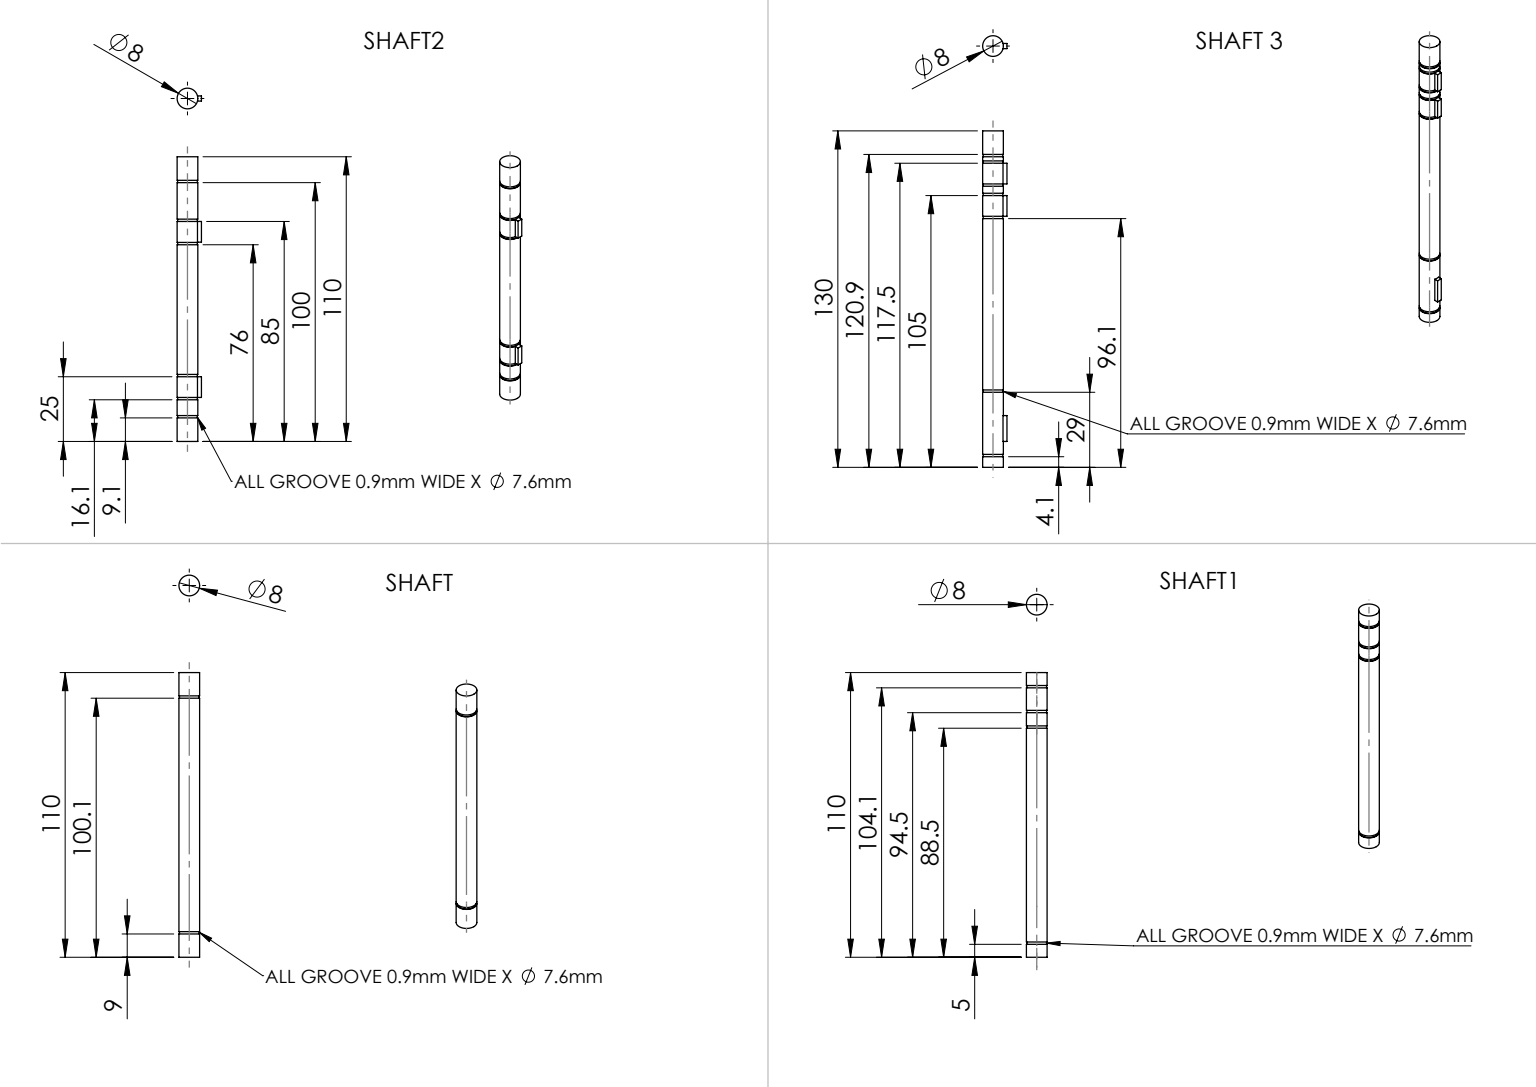
ISO-10303-21;
HEADER;
FILE_DESCRIPTION (('STEP AP214'),
    '1' );
FILE_NAME ('shaft 3.step',
    '2026-09-28T15:49:00',
    ( '' ),
    ( '' ),
    'SwSTEP 2.0',
    'SolidWorks 2026',
    '' );
FILE_SCHEMA (( 'AUTOMOTIVE_DESIGN' ));
ENDSEC;

DATA;
#35=DIRECTION ( 'NONE',  ( 0.000000000000000000, 0.000000000000000000, 1.000000000000000000 ) ) ;
#45=CIRCLE ( 'NONE', #32841, 4.000000000000000000 ) ;
#49=ORIENTED_EDGE ( 'NONE', *, *, #14010, .T. ) ;
#53=ORIENTED_EDGE ( 'NONE', *, *, #22089, .T. ) ;
#63=EDGE_CURVE ( 'NONE', #29341, #31925, #15789, .T. ) ;
#64=FACE_BOUND ( 'NONE', #18708, .T. ) ;
#78=CARTESIAN_POINT ( 'NONE',  ( 0.000000000000000000, 0.000000000000000000, -52.50000000000000000 ) ) ;
#94=EDGE_LOOP ( 'NONE', ( #19216, #26930 ) ) ;
#103=DIRECTION ( 'NONE',  ( 0.000000000000000000, 0.000000000000000000, 1.000000000000000000 ) ) ;
#158=DIRECTION ( 'NONE',  ( 1.000000000000000000, 0.000000000000000000, 0.000000000000000000 ) ) ;
#161=AXIS2_PLACEMENT_3D ( 'NONE', #25822, #31910, #29039 ) ;
#163=AXIS2_PLACEMENT_3D ( 'NONE', #32400, #32750, #18355 ) ;
#170=EDGE_LOOP ( 'NONE', ( #28975, #27946, #5714, #16850, #18978 ) ) ;
#184=ORIENTED_EDGE ( 'NONE', *, *, #5407, .T. ) ;
#201=DIRECTION ( 'NONE',  ( 0.000000000000000000, 0.000000000000000000, -1.000000000000000000 ) ) ;
#243=UNCERTAINTY_MEASURE_WITH_UNIT (LENGTH_MEASURE( 1.000000000000000082E-05 ), #22968, 'distance_accuracy_value', 'NONE');
#244=FACE_BOUND ( 'NONE', #10635, .T. ) ;
#313=EDGE_CURVE ( 'NONE', #20125, #14882, #23736, .T. ) ;
#334=VERTEX_POINT ( 'NONE', #10530 ) ;
#363=VECTOR ( 'NONE', #32529, 1000.000000000000000 ) ;
#379=CIRCLE ( 'NONE', #19345, 3.799999999999999822 ) ;
#397=VECTOR ( 'NONE', #13640, 1000.000000000000000 ) ;
#407=ORIENTED_EDGE ( 'NONE', *, *, #33311, .T. ) ;
#422=AXIS2_PLACEMENT_3D ( 'NONE', #13815, #3025, #22085 ) ;
#445=ORIENTED_EDGE ( 'NONE', *, *, #2012, .T. ) ;
#457=AXIS2_PLACEMENT_3D ( 'NONE', #23375, #28612, #18143 ) ;
#529=VERTEX_POINT ( 'NONE', #3676 ) ;
#548=DIRECTION ( 'NONE',  ( 0.000000000000000000, 0.000000000000000000, -1.000000000000000000 ) ) ;
#559=CARTESIAN_POINT ( 'NONE',  ( 0.000000000000000000, 0.000000000000000000, 36.00000000000000000 ) ) ;
#569=ORIENTED_EDGE ( 'NONE', *, *, #1551, .F. ) ;
#602=AXIS2_PLACEMENT_3D ( 'NONE', #22892, #9216, #15491 ) ;
#667=EDGE_CURVE ( 'NONE', #19003, #35092, #26350, .T. ) ;
#681=ADVANCED_FACE ( 'NONE', ( #6712 ), #12122, .T. ) ;
#708=VERTEX_POINT ( 'NONE', #10129 ) ;
#719=FACE_BOUND ( 'NONE', #18642, .T. ) ;
#759=EDGE_CURVE ( 'NONE', #1825, #2615, #29234, .T. ) ;
#762=EDGE_LOOP ( 'NONE', ( #23017, #33225, #3692, #5978 ) ) ;
#799=AXIS2_PLACEMENT_3D ( 'NONE', #2899, #3428, #30949 ) ;
#875=DIRECTION ( 'NONE',  ( -1.000000000000000000, 0.000000000000000000, 0.000000000000000000 ) ) ;
#891=VERTEX_POINT ( 'NONE', #10669 ) ;
#925=EDGE_CURVE ( 'NONE', #1732, #8675, #21625, .T. ) ;
#926=ADVANCED_FACE ( 'NONE', ( #19110 ), #21813, .F. ) ;
#939=DIRECTION ( 'NONE',  ( 0.000000000000000000, 0.000000000000000000, -1.000000000000000000 ) ) ;
#946=VECTOR ( 'NONE', #32460, 1000.000000000000000 ) ;
#971=CARTESIAN_POINT ( 'NONE',  ( -4.000000000000000000, 0.000000000000000000, 65.00000000000000000 ) ) ;
#1057=AXIS2_PLACEMENT_3D ( 'NONE', #25207, #11856, #34016 ) ;
#1062=CARTESIAN_POINT ( 'NONE',  ( -4.000000000000000000, 0.000000000000000000, -40.00000000000000711 ) ) ;
#1089=EDGE_CURVE ( 'NONE', #18547, #14157, #25484, .T. ) ;
#1104=EDGE_CURVE ( 'NONE', #9474, #16728, #8811, .T. ) ;
#1115=CARTESIAN_POINT ( 'NONE',  ( 4.000000000000000000, 4.898587196589412829E-16, 55.00000000000000711 ) ) ;
#1131=ORIENTED_EDGE ( 'NONE', *, *, #8517, .T. ) ;
#1185=EDGE_LOOP ( 'NONE', ( #21946, #29122, #4099, #24705 ) ) ;
#1199=ORIENTED_EDGE ( 'NONE', *, *, #32627, .T. ) ;
#1200=ORIENTED_EDGE ( 'NONE', *, *, #17363, .T. ) ;
#1212=FACE_BOUND ( 'NONE', #25738, .T. ) ;
#1243=PLANE ( 'NONE',  #13482 ) ;
#1250=DIRECTION ( 'NONE',  ( 1.000000000000000000, 0.000000000000000000, 0.000000000000000000 ) ) ;
#1290=FACE_OUTER_BOUND ( 'NONE', #13785, .T. ) ;
#1308=CARTESIAN_POINT ( 'NONE',  ( 5.400000000000085620, -1.000000000000049516, -44.50000000000000000 ) ) ;
#1386=ADVANCED_FACE ( 'NONE', ( #10817 ), #35486, .F. ) ;
#1408=LINE ( 'NONE', #20464, #3158 ) ;
#1411=DIRECTION ( 'NONE',  ( 1.000000000000000000, 0.000000000000000000, 0.000000000000000000 ) ) ;
#1422=ORIENTED_EDGE ( 'NONE', *, *, #667, .F. ) ;
#1425=CARTESIAN_POINT ( 'NONE',  ( 0.000000000000000000, 0.000000000000000000, -53.39999999999999858 ) ) ;
#1483=AXIS2_PLACEMENT_3D ( 'NONE', #27788, #939, #24901 ) ;
#1511=LINE ( 'NONE', #12493, #7664 ) ;
#1546=VERTEX_POINT ( 'NONE', #35138 ) ;
#1551=EDGE_CURVE ( 'NONE', #20125, #33416, #27029, .T. ) ;
#1555=CARTESIAN_POINT ( 'NONE',  ( 9.714451465470119729E-14, 0.9999999999999870104, -52.50000000000000000 ) ) ;
#1570=CARTESIAN_POINT ( 'NONE',  ( 3.799999999999999822, 0.000000000000000000, -43.60000000000000142 ) ) ;
#1604=DIRECTION ( 'NONE',  ( -1.000000000000000000, 1.110223024625156540E-16, 0.000000000000000000 ) ) ;
#1608=VECTOR ( 'NONE', #26480, 1000.000000000000000 ) ;
#1627=ADVANCED_FACE ( 'NONE', ( #16893 ), #33129, .T. ) ;
#1680=CARTESIAN_POINT ( 'NONE',  ( 0.000000000000000000, 0.000000000000000000, -44.50000000000000000 ) ) ;
#1708=EDGE_CURVE ( 'NONE', #10690, #33549, #14030, .T. ) ;
#1726=PLANE ( 'NONE',  #34542 ) ;
#1732=VERTEX_POINT ( 'NONE', #11857 ) ;
#1792=ADVANCED_FACE ( 'NONE', ( #15077 ), #1243, .F. ) ;
#1804=CARTESIAN_POINT ( 'NONE',  ( 0.000000000000000000, 0.000000000000000000, -65.00000000000000000 ) ) ;
#1825=VERTEX_POINT ( 'NONE', #31305 ) ;
#1844=( NAMED_UNIT ( * ) SI_UNIT ( $, .STERADIAN. ) SOLID_ANGLE_UNIT ( ) );
#1850=VERTEX_POINT ( 'NONE', #26266 ) ;
#1869=CIRCLE ( 'NONE', #16244, 4.000000000000000000 ) ;
#1889=DIRECTION ( 'NONE',  ( 0.000000000000000000, 0.000000000000000000, 1.000000000000000000 ) ) ;
#1939=DIRECTION ( 'NONE',  ( -1.000000000000000000, 0.000000000000000000, 0.000000000000000000 ) ) ;
#1949=DIRECTION ( 'NONE',  ( 0.000000000000000000, 0.000000000000000000, 1.000000000000000000 ) ) ;
#1997=EDGE_CURVE ( 'NONE', #15000, #23250, #32199, .T. ) ;
#2012=EDGE_CURVE ( 'NONE', #5174, #9474, #13646, .T. ) ;
#2210=VERTEX_POINT ( 'NONE', #8932 ) ;
#2215=ORIENTED_EDGE ( 'NONE', *, *, #19628, .T. ) ;
#2274=CARTESIAN_POINT ( 'NONE',  ( -3.799999999999999822, 4.653657836759942730E-16, 36.00000000000000000 ) ) ;
#2286=ADVANCED_FACE ( 'NONE', ( #20615 ), #34149, .T. ) ;
#2290=CYLINDRICAL_SURFACE ( 'NONE', #32641, 4.000000000000000000 ) ;
#2299=FACE_OUTER_BOUND ( 'NONE', #28981, .T. ) ;
#2300=EDGE_CURVE ( 'NONE', #17838, #10539, #13512, .T. ) ;
#2305=EDGE_LOOP ( 'NONE', ( #16724, #26388, #32363, #12762 ) ) ;
#2311=AXIS2_PLACEMENT_3D ( 'NONE', #28801, #12776, #4327 ) ;
#2355=VECTOR ( 'NONE', #11953, 1000.000000000000000 ) ;
#2357=DIRECTION ( 'NONE',  ( -1.000000000000000000, 0.000000000000000000, 0.000000000000000000 ) ) ;
#2394=CIRCLE ( 'NONE', #19595, 4.000000000000000000 ) ;
#2432=CARTESIAN_POINT ( 'NONE',  ( -4.000000000000000000, 0.000000000000000000, -40.89999999999999858 ) ) ;
#2504=VERTEX_POINT ( 'NONE', #21694 ) ;
#2506=EDGE_LOOP ( 'NONE', ( #10673, #1199, #407, #34930 ) ) ;
#2513=ORIENTED_EDGE ( 'NONE', *, *, #34592, .F. ) ;
#2528=CARTESIAN_POINT ( 'NONE',  ( 5.400000000000085620, -1.000000000000049516, -32.00000000000000000 ) ) ;
#2537=ORIENTED_EDGE ( 'NONE', *, *, #1089, .T. ) ;
#2547=AXIS2_PLACEMENT_3D ( 'NONE', #16252, #21483, #32476 ) ;
#2576=AXIS2_PLACEMENT_3D ( 'NONE', #11160, #33643, #875 ) ;
#2603=DIRECTION ( 'NONE',  ( -0.000000000000000000, 0.000000000000000000, -1.000000000000000000 ) ) ;
#2615=VERTEX_POINT ( 'NONE', #16277 ) ;
#2620=DIRECTION ( 'NONE',  ( -1.000000000000000000, 0.000000000000000000, 0.000000000000000000 ) ) ;
#2656=AXIS2_PLACEMENT_3D ( 'NONE', #3682, #14632, #19675 ) ;
#2665=AXIS2_PLACEMENT_3D ( 'NONE', #16709, #18893, #16351 ) ;
#2674=LINE ( 'NONE', #29500, #397 ) ;
#2693=VERTEX_POINT ( 'NONE', #11083 ) ;
#2738=ORIENTED_EDGE ( 'NONE', *, *, #27732, .F. ) ;
#2790=LINE ( 'NONE', #12548, #11992 ) ;
#2792=DIRECTION ( 'NONE',  ( -1.000000000000000000, 0.000000000000000000, 0.000000000000000000 ) ) ;
#2793=AXIS2_PLACEMENT_3D ( 'NONE', #9523, #6992, #31309 ) ;
#2847=DIRECTION ( 'NONE',  ( -1.000000000000000000, 0.000000000000000000, 0.000000000000000000 ) ) ;
#2899=CARTESIAN_POINT ( 'NONE',  ( 0.000000000000000000, 0.000000000000000000, -40.89999999999999858 ) ) ;
#2901=EDGE_CURVE ( 'NONE', #13424, #2693, #1511, .T. ) ;
#2935=DIRECTION ( 'NONE',  ( -1.000000000000000000, 0.000000000000000000, 0.000000000000000000 ) ) ;
#3018=DIRECTION ( 'NONE',  ( 1.000000000000000000, -1.110223024625156540E-16, 0.000000000000000000 ) ) ;
#3025=DIRECTION ( 'NONE',  ( 1.110223024625156540E-16, 1.000000000000000000, 0.000000000000000000 ) ) ;
#3048=AXIS2_PLACEMENT_3D ( 'NONE', #11758, #3330, #33731 ) ;
#3086=AXIS2_PLACEMENT_3D ( 'NONE', #9014, #22341, #11712 ) ;
#3125=ORIENTED_EDGE ( 'NONE', *, *, #31259, .T. ) ;
#3136=DIRECTION ( 'NONE',  ( -1.000000000000000000, 8.604228440844963188E-16, 0.000000000000000000 ) ) ;
#3158=VECTOR ( 'NONE', #26077, 1000.000000000000000 ) ;
#3196=PLANE ( 'NONE',  #422 ) ;
#3243=FACE_OUTER_BOUND ( 'NONE', #27570, .T. ) ;
#3268=DIRECTION ( 'NONE',  ( -0.000000000000000000, 0.000000000000000000, -1.000000000000000000 ) ) ;
#3282=VERTEX_POINT ( 'NONE', #30098 ) ;
#3311=AXIS2_PLACEMENT_3D ( 'NONE', #78, #11065, #22035 ) ;
#3328=ADVANCED_FACE ( 'NONE', ( #24167 ), #16388, .T. ) ;
#3330=DIRECTION ( 'NONE',  ( 0.000000000000000000, 0.000000000000000000, -1.000000000000000000 ) ) ;
#3339=CARTESIAN_POINT ( 'NONE',  ( 0.000000000000000000, 0.000000000000000000, 60.90000000000001279 ) ) ;
#3373=CARTESIAN_POINT ( 'NONE',  ( 1.110223024625156540E-13, -1.000000000000042633, -52.50000000000000000 ) ) ;
#3393=PLANE ( 'NONE',  #18283 ) ;
#3400=CYLINDRICAL_SURFACE ( 'NONE', #16840, 4.000000000000000000 ) ;
#3428=DIRECTION ( 'NONE',  ( 0.000000000000000000, 0.000000000000000000, 1.000000000000000000 ) ) ;
#3431=AXIS2_PLACEMENT_3D ( 'NONE', #3458, #30804, #5797 ) ;
#3458=CARTESIAN_POINT ( 'NONE',  ( 0.000000000000000000, 0.000000000000000000, -31.10000000000000142 ) ) ;
#3492=CARTESIAN_POINT ( 'NONE',  ( 3.872983346207517386, -1.000000000000028644, -40.00000000000000711 ) ) ;
#3507=DIRECTION ( 'NONE',  ( -1.000000000000000000, 0.000000000000000000, 0.000000000000000000 ) ) ;
#3549=CARTESIAN_POINT ( 'NONE',  ( 5.400000000000085620, -1.000000000000049516, -32.00000000000000000 ) ) ;
#3558=CARTESIAN_POINT ( 'NONE',  ( -3.799999999999999822, 4.653657836759942730E-16, -40.89999999999999858 ) ) ;
#3580=DIRECTION ( 'NONE',  ( 0.000000000000000000, 0.000000000000000000, -1.000000000000000000 ) ) ;
#3619=AXIS2_PLACEMENT_3D ( 'NONE', #31515, #15279, #17807 ) ;
#3643=ORIENTED_EDGE ( 'NONE', *, *, #15823, .T. ) ;
#3649=ORIENTED_EDGE ( 'NONE', *, *, #4897, .F. ) ;
#3659=EDGE_CURVE ( 'NONE', #32739, #28967, #8206, .T. ) ;
#3669=CARTESIAN_POINT ( 'NONE',  ( 0.000000000000000000, 0.000000000000000000, -53.39999999999999858 ) ) ;
#3676=CARTESIAN_POINT ( 'NONE',  ( 3.799999999999999822, 0.000000000000000000, -53.39999999999999858 ) ) ;
#3682=CARTESIAN_POINT ( 'NONE',  ( 0.000000000000000000, 0.000000000000000000, 60.00000000000000000 ) ) ;
#3687=DIRECTION ( 'NONE',  ( 0.000000000000000000, 0.000000000000000000, -1.000000000000000000 ) ) ;
#3692=ORIENTED_EDGE ( 'NONE', *, *, #7492, .T. ) ;
#3716=VECTOR ( 'NONE', #9190, 1000.000000000000000 ) ;
#3753=CARTESIAN_POINT ( 'NONE',  ( 0.000000000000000000, 0.000000000000000000, -44.50000000000000000 ) ) ;
#3771=CARTESIAN_POINT ( 'NONE',  ( 3.872983346207517386, -1.000000000000028644, 65.00000000000000000 ) ) ;
#3772=CIRCLE ( 'NONE', #11790, 4.000000000000000000 ) ;
#3777=CIRCLE ( 'NONE', #1483, 3.799999999999999822 ) ;
#3790=CARTESIAN_POINT ( 'NONE',  ( 3.872983346207517386, -1.000000000000028644, 45.00000000000000711 ) ) ;
#3805=FACE_OUTER_BOUND ( 'NONE', #2506, .T. ) ;
#3818=ADVANCED_FACE ( 'NONE', ( #32047 ), #18887, .T. ) ;
#3840=AXIS2_PLACEMENT_3D ( 'NONE', #18949, #10329, #35538 ) ;
#3900=CIRCLE ( 'NONE', #3311, 4.000000000000000000 ) ;
#3912=VECTOR ( 'NONE', #31497, 1000.000000000000000 ) ;
#3917=LINE ( 'NONE', #1555, #26870 ) ;
#3965=AXIS2_PLACEMENT_3D ( 'NONE', #10553, #103, #30006 ) ;
#3992=FACE_OUTER_BOUND ( 'NONE', #30123, .T. ) ;
#3997=VERTEX_POINT ( 'NONE', #30578 ) ;
#4033=DIRECTION ( 'NONE',  ( 0.000000000000000000, 0.000000000000000000, -1.000000000000000000 ) ) ;
#4042=PLANE ( 'NONE',  #23335 ) ;
#4046=AXIS2_PLACEMENT_3D ( 'NONE', #8922, #31077, #28028 ) ;
#4050=FACE_OUTER_BOUND ( 'NONE', #30940, .T. ) ;
#4069=ADVANCED_FACE ( 'NONE', ( #9499 ), #28946, .T. ) ;
#4099=ORIENTED_EDGE ( 'NONE', *, *, #1997, .F. ) ;
#4129=FACE_BOUND ( 'NONE', #21760, .T. ) ;
#4166=DIRECTION ( 'NONE',  ( -0.000000000000000000, 0.000000000000000000, -1.000000000000000000 ) ) ;
#4224=DIRECTION ( 'NONE',  ( 0.000000000000000000, 0.000000000000000000, -1.000000000000000000 ) ) ;
#4255=CARTESIAN_POINT ( 'NONE',  ( 0.000000000000000000, 0.000000000000000000, 60.00000000000000000 ) ) ;
#4281=EDGE_CURVE ( 'NONE', #11309, #17651, #27314, .T. ) ;
#4312=CARTESIAN_POINT ( 'NONE',  ( 1.110223024625156540E-13, -1.000000000000042633, -44.50000000000000000 ) ) ;
#4317=DIRECTION ( 'NONE',  ( -0.000000000000000000, 0.000000000000000000, -1.000000000000000000 ) ) ;
#4327=DIRECTION ( 'NONE',  ( -1.000000000000000000, 0.000000000000000000, 0.000000000000000000 ) ) ;
#4366=ORIENTED_EDGE ( 'NONE', *, *, #16719, .F. ) ;
#4389=CARTESIAN_POINT ( 'NONE',  ( 0.000000000000000000, 0.000000000000000000, -40.89999999999999858 ) ) ;
#4431=CIRCLE ( 'NONE', #11305, 3.799999999999999822 ) ;
#4439=LINE ( 'NONE', #10182, #11323 ) ;
#4440=CARTESIAN_POINT ( 'NONE',  ( 0.000000000000000000, 0.000000000000000000, -40.00000000000000000 ) ) ;
#4465=DIRECTION ( 'NONE',  ( 0.000000000000000000, 0.000000000000000000, -1.000000000000000000 ) ) ;
#4475=DIRECTION ( 'NONE',  ( 0.000000000000000000, 0.000000000000000000, -1.000000000000000000 ) ) ;
#4477=VECTOR ( 'NONE', #3136, 1000.000000000000000 ) ;
#4527=DIRECTION ( 'NONE',  ( 0.000000000000000000, 0.000000000000000000, -1.000000000000000000 ) ) ;
#4531=FACE_OUTER_BOUND ( 'NONE', #15351, .T. ) ;
#4558=PRESENTATION_STYLE_ASSIGNMENT (( #26863 ) ) ;
#4630=( NAMED_UNIT ( * ) PLANE_ANGLE_UNIT ( ) SI_UNIT ( $, .RADIAN. ) );
#4645=ORIENTED_EDGE ( 'NONE', *, *, #28476, .T. ) ;
#4652=ORIENTED_EDGE ( 'NONE', *, *, #24673, .F. ) ;
#4663=FACE_OUTER_BOUND ( 'NONE', #2305, .T. ) ;
#4666=CARTESIAN_POINT ( 'NONE',  ( 0.000000000000000000, 0.000000000000000000, -40.89999999999999858 ) ) ;
#4729=ORIENTED_EDGE ( 'NONE', *, *, #30126, .T. ) ;
#4736=ADVANCED_FACE ( 'NONE', ( #22032, #11708 ), #14405, .F. ) ;
#4777=CARTESIAN_POINT ( 'NONE',  ( -4.000000000000000000, 0.000000000000000000, -55.89999999999999858 ) ) ;
#4845=EDGE_CURVE ( 'NONE', #12683, #2615, #22867, .T. ) ;
#4852=ADVANCED_FACE ( 'NONE', ( #27098, #13408 ), #35376, .T. ) ;
#4853=LINE ( 'NONE', #12947, #8691 ) ;
#4884=ADVANCED_FACE ( 'NONE', ( #3992, #23044 ), #14763, .F. ) ;
#4897=EDGE_CURVE ( 'NONE', #28967, #28820, #17816, .T. ) ;
#4898=SURFACE_SIDE_STYLE ('',( #29384 ) ) ;
#4910=AXIS2_PLACEMENT_3D ( 'NONE', #32006, #7345, #24099 ) ;
#4920=ORIENTED_EDGE ( 'NONE', *, *, #2300, .T. ) ;
#5004=AXIS2_PLACEMENT_3D ( 'NONE', #22998, #3580, #14527 ) ;
#5037=ORIENTED_EDGE ( 'NONE', *, *, #17189, .F. ) ;
#5096=VECTOR ( 'NONE', #8374, 1000.000000000000000 ) ;
#5108=ADVANCED_FACE ( 'NONE', ( #5235 ), #21049, .T. ) ;
#5174=VERTEX_POINT ( 'NONE', #22297 ) ;
#5175=AXIS2_PLACEMENT_3D ( 'NONE', #17449, #14748, #18525 ) ;
#5191=CYLINDRICAL_SURFACE ( 'NONE', #29029, 3.799999999999999822 ) ;
#5205=CARTESIAN_POINT ( 'NONE',  ( -3.799999999999999822, 4.653657836759942730E-16, 35.10000000000000142 ) ) ;
#5235=FACE_OUTER_BOUND ( 'NONE', #33749, .T. ) ;
#5242=ORIENTED_EDGE ( 'NONE', *, *, #16113, .T. ) ;
#5263=DIRECTION ( 'NONE',  ( 1.000000000000000000, 0.000000000000000000, 0.000000000000000000 ) ) ;
#5276=DIRECTION ( 'NONE',  ( 1.000000000000000000, 0.000000000000000000, 0.000000000000000000 ) ) ;
#5277=CIRCLE ( 'NONE', #12147, 4.000000000000000000 ) ;
#5282=VERTEX_POINT ( 'NONE', #19582 ) ;
#5286=DIRECTION ( 'NONE',  ( 0.000000000000000000, 0.000000000000000000, -1.000000000000000000 ) ) ;
#5304=LINE ( 'NONE', #16242, #22925 ) ;
#5329=VERTEX_POINT ( 'NONE', #17237 ) ;
#5361=LINE ( 'NONE', #15961, #21056 ) ;
#5362=DIRECTION ( 'NONE',  ( 0.000000000000000000, 0.000000000000000000, -1.000000000000000000 ) ) ;
#5371=ORIENTED_EDGE ( 'NONE', *, *, #14296, .T. ) ;
#5383=CARTESIAN_POINT ( 'NONE',  ( 9.714451465470119729E-14, 0.9999999999999870104, -32.00000000000000000 ) ) ;
#5407=EDGE_CURVE ( 'NONE', #23250, #34581, #1408, .T. ) ;
#5421=AXIS2_PLACEMENT_3D ( 'NONE', #21421, #16185, #29553 ) ;
#5498=EDGE_CURVE ( 'NONE', #21576, #30905, #34005, .T. ) ;
#5512=CARTESIAN_POINT ( 'NONE',  ( 3.799999999999999822, 0.000000000000000000, 60.90000000000001279 ) ) ;
#5528=CYLINDRICAL_SURFACE ( 'NONE', #18245, 3.799999999999999822 ) ;
#5559=ADVANCED_FACE ( 'NONE', ( #10576 ), #5191, .T. ) ;
#5604=CARTESIAN_POINT ( 'NONE',  ( 0.000000000000000000, 0.000000000000000000, 55.00000000000000711 ) ) ;
#5616=EDGE_CURVE ( 'NONE', #32249, #2504, #3772, .T. ) ;
#5652=EDGE_CURVE ( 'NONE', #28820, #8675, #32488, .T. ) ;
#5653=CIRCLE ( 'NONE', #32659, 3.799999999999999822 ) ;
#5692=DIRECTION ( 'NONE',  ( 1.000000000000000000, 0.000000000000000000, 0.000000000000000000 ) ) ;
#5695=ADVANCED_FACE ( 'NONE', ( #13120 ), #21003, .T. ) ;
#5708=EDGE_LOOP ( 'NONE', ( #10243, #32904 ) ) ;
#5714=ORIENTED_EDGE ( 'NONE', *, *, #22916, .T. ) ;
#5738=EDGE_CURVE ( 'NONE', #19012, #12683, #8390, .T. ) ;
#5744=CARTESIAN_POINT ( 'NONE',  ( 0.000000000000000000, 0.000000000000000000, -40.00000000000000000 ) ) ;
#5797=DIRECTION ( 'NONE',  ( -1.000000000000000000, 0.000000000000000000, 0.000000000000000000 ) ) ;
#5873=CYLINDRICAL_SURFACE ( 'NONE', #18776, 4.000000000000000000 ) ;
#5913=DIRECTION ( 'NONE',  ( -1.000000000000000000, 0.000000000000000000, 0.000000000000000000 ) ) ;
#5944=EDGE_LOOP ( 'NONE', ( #18134, #30778, #21079, #31987 ) ) ;
#5962=EDGE_CURVE ( 'NONE', #21809, #12683, #34496, .T. ) ;
#5978=ORIENTED_EDGE ( 'NONE', *, *, #10678, .T. ) ;
#5985=ORIENTED_EDGE ( 'NONE', *, *, #14960, .F. ) ;
#6061=DIRECTION ( 'NONE',  ( 0.000000000000000000, 0.000000000000000000, 1.000000000000000000 ) ) ;
#6063=AXIS2_PLACEMENT_3D ( 'NONE', #6140, #4166, #11888 ) ;
#6065=UNCERTAINTY_MEASURE_WITH_UNIT (LENGTH_MEASURE( 1.000000000000000082E-05 ), #29911, 'distance_accuracy_value', 'NONE');
#6072=SHAPE_DEFINITION_REPRESENTATION ( #23625, #18063 ) ;
#6103=ORIENTED_EDGE ( 'NONE', *, *, #1104, .T. ) ;
#6132=FACE_OUTER_BOUND ( 'NONE', #18192, .T. ) ;
#6140=CARTESIAN_POINT ( 'NONE',  ( 0.000000000000000000, 0.000000000000000000, 65.00000000000000000 ) ) ;
#6154=EDGE_CURVE ( 'NONE', #708, #12699, #9517, .T. ) ;
#6303=CARTESIAN_POINT ( 'NONE',  ( 0.000000000000000000, 0.000000000000000000, 65.00000000000000000 ) ) ;
#6315=ORIENTED_EDGE ( 'NONE', *, *, #25365, .T. ) ;
#6317=DIRECTION ( 'NONE',  ( 0.000000000000000000, 0.000000000000000000, -1.000000000000000000 ) ) ;
#6338=ORIENTED_EDGE ( 'NONE', *, *, #9978, .T. ) ;
#6342=PRODUCT ( 'shaft 3', 'shaft 3', '', ( #30737 ) ) ;
#6387=CARTESIAN_POINT ( 'NONE',  ( 0.000000000000000000, 0.000000000000000000, -43.60000000000000142 ) ) ;
#6419=EDGE_CURVE ( 'NONE', #529, #334, #20198, .T. ) ;
#6444=DIRECTION ( 'NONE',  ( 1.000000000000000000, -1.110223024625156540E-16, 0.000000000000000000 ) ) ;
#6473=ORIENTED_EDGE ( 'NONE', *, *, #2901, .T. ) ;
#6487=DIRECTION ( 'NONE',  ( -1.000000000000000000, 0.000000000000000000, 0.000000000000000000 ) ) ;
#6515=PRODUCT_DEFINITION_CONTEXT ( 'detailed design', #19717, 'design' ) ;
#6520=ADVANCED_FACE ( 'NONE', ( #22737, #33732 ), #4042, .T. ) ;
#6525=CARTESIAN_POINT ( 'NONE',  ( 5.400000000000085620, -1.000000000000049516, -40.00000000000000000 ) ) ;
#6550=ORIENTED_EDGE ( 'NONE', *, *, #29747, .T. ) ;
#6577=ORIENTED_EDGE ( 'NONE', *, *, #31132, .T. ) ;
#6589=ADVANCED_FACE ( 'NONE', ( #13024, #24013 ), #18409, .F. ) ;
#6614=EDGE_CURVE ( 'NONE', #8976, #12699, #21282, .T. ) ;
#6646=EDGE_LOOP ( 'NONE', ( #7286, #1200 ) ) ;
#6675=PLANE ( 'NONE',  #19605 ) ;
#6712=FACE_OUTER_BOUND ( 'NONE', #31261, .T. ) ;
#6718=LINE ( 'NONE', #971, #2355 ) ;
#6740=AXIS2_PLACEMENT_3D ( 'NONE', #34703, #24254, #1939 ) ;
#6741=VECTOR ( 'NONE', #27815, 1000.000000000000000 ) ;
#6804=PLANE ( 'NONE',  #19326 ) ;
#6847=PRODUCT_DEFINITION ( 'UNKNOWN', '', #18955, #6515 ) ;
#6853=ORIENTED_EDGE ( 'NONE', *, *, #14960, .T. ) ;
#6945=DIRECTION ( 'NONE',  ( -0.000000000000000000, 0.000000000000000000, -1.000000000000000000 ) ) ;
#6946=ORIENTED_EDGE ( 'NONE', *, *, #34786, .F. ) ;
#6947=ORIENTED_EDGE ( 'NONE', *, *, #18970, .F. ) ;
#6963=FACE_OUTER_BOUND ( 'NONE', #10244, .T. ) ;
#6968=EDGE_CURVE ( 'NONE', #3997, #31797, #8989, .T. ) ;
#6992=DIRECTION ( 'NONE',  ( 0.000000000000000000, 0.000000000000000000, -1.000000000000000000 ) ) ;
#6994=AXIS2_PLACEMENT_3D ( 'NONE', #13711, #8112, #5263 ) ;
#7025=AXIS2_PLACEMENT_3D ( 'NONE', #8370, #24606, #5692 ) ;
#7027=EDGE_LOOP ( 'NONE', ( #15396, #22436, #15486, #19299 ) ) ;
#7036=DIRECTION ( 'NONE',  ( -1.000000000000000000, 0.000000000000000000, 0.000000000000000000 ) ) ;
#7066=DIRECTION ( 'NONE',  ( 0.000000000000000000, 0.000000000000000000, -1.000000000000000000 ) ) ;
#7094=AXIS2_PLACEMENT_3D ( 'NONE', #13729, #24008, #32808 ) ;
#7156=CARTESIAN_POINT ( 'NONE',  ( -3.799999999999999822, 4.653657836759942730E-16, -32.00000000000000000 ) ) ;
#7158=LINE ( 'NONE', #23728, #363 ) ;
#7177=DIRECTION ( 'NONE',  ( 0.000000000000000000, 0.000000000000000000, 1.000000000000000000 ) ) ;
#7276=AXIS2_PLACEMENT_3D ( 'NONE', #10076, #21231, #2357 ) ;
#7286=ORIENTED_EDGE ( 'NONE', *, *, #27833, .T. ) ;
#7298=DIRECTION ( 'NONE',  ( -1.000000000000000000, 1.110223024625156540E-16, 0.000000000000000000 ) ) ;
#7333=CARTESIAN_POINT ( 'NONE',  ( 0.000000000000000000, 0.000000000000000000, -43.60000000000000142 ) ) ;
#7345=DIRECTION ( 'NONE',  ( 1.110223024625156540E-16, 1.000000000000000000, 0.000000000000000000 ) ) ;
#7359=ORIENTED_EDGE ( 'NONE', *, *, #27347, .F. ) ;
#7375=ORIENTED_EDGE ( 'NONE', *, *, #21969, .F. ) ;
#7414=ORIENTED_EDGE ( 'NONE', *, *, #19628, .F. ) ;
#7430=ORIENTED_EDGE ( 'NONE', *, *, #14341, .T. ) ;
#7492=EDGE_CURVE ( 'NONE', #14157, #28884, #13233, .T. ) ;
#7515=VERTEX_POINT ( 'NONE', #2432 ) ;
#7559=ORIENTED_EDGE ( 'NONE', *, *, #925, .F. ) ;
#7584=VERTEX_POINT ( 'NONE', #27629 ) ;
#7602=DIRECTION ( 'NONE',  ( 0.000000000000000000, 0.000000000000000000, -1.000000000000000000 ) ) ;
#7605=ORIENTED_EDGE ( 'NONE', *, *, #31891, .F. ) ;
#7652=CARTESIAN_POINT ( 'NONE',  ( 4.000000000000000000, 4.898587196589412829E-16, -31.10000000000000142 ) ) ;
#7664=VECTOR ( 'NONE', #23475, 1000.000000000000000 ) ;
#7665=CARTESIAN_POINT ( 'NONE',  ( -4.000000000000000000, 0.000000000000000000, -43.60000000000000142 ) ) ;
#7669=CARTESIAN_POINT ( 'NONE',  ( 3.872983346207489852, 0.9999999999999522604, 65.00000000000000000 ) ) ;
#7693=DIRECTION ( 'NONE',  ( 0.000000000000000000, 0.000000000000000000, 1.000000000000000000 ) ) ;
#7750=EDGE_CURVE ( 'NONE', #1850, #10066, #30322, .T. ) ;
#7773=DIRECTION ( 'NONE',  ( -0.000000000000000000, 0.000000000000000000, -1.000000000000000000 ) ) ;
#7777=DIRECTION ( 'NONE',  ( 0.000000000000000000, 0.000000000000000000, -1.000000000000000000 ) ) ;
#7816=VECTOR ( 'NONE', #23457, 1000.000000000000000 ) ;
#7879=( GEOMETRIC_REPRESENTATION_CONTEXT ( 3 ) GLOBAL_UNCERTAINTY_ASSIGNED_CONTEXT ( ( #243 ) ) GLOBAL_UNIT_ASSIGNED_CONTEXT ( ( #22968, #4630, #23150 ) ) REPRESENTATION_CONTEXT ( 'NONE', 'WORKASPACE' ) );
#7906=CARTESIAN_POINT ( 'NONE',  ( 5.400000000000085620, -1.000000000000049516, -52.50000000000000000 ) ) ;
#8041=FACE_OUTER_BOUND ( 'NONE', #10730, .T. ) ;
#8052=ORIENTED_EDGE ( 'NONE', *, *, #33644, .T. ) ;
#8081=CARTESIAN_POINT ( 'NONE',  ( 0.000000000000000000, 0.000000000000000000, 60.90000000000001279 ) ) ;
#8083=DIRECTION ( 'NONE',  ( 0.000000000000000000, 0.000000000000000000, 1.000000000000000000 ) ) ;
#8096=EDGE_LOOP ( 'NONE', ( #29389, #28425, #12580, #34605 ) ) ;
#8112=DIRECTION ( 'NONE',  ( 0.000000000000000000, 0.000000000000000000, 1.000000000000000000 ) ) ;
#8125=ORIENTED_EDGE ( 'NONE', *, *, #34786, .T. ) ;
#8129=DIRECTION ( 'NONE',  ( -0.000000000000000000, 0.000000000000000000, -1.000000000000000000 ) ) ;
#8198=ORIENTED_EDGE ( 'NONE', *, *, #759, .T. ) ;
#8206=CIRCLE ( 'NONE', #3619, 4.000000000000000000 ) ;
#8212=CARTESIAN_POINT ( 'NONE',  ( 3.872983346207517386, -1.000000000000028644, 55.00000000000000711 ) ) ;
#8225=DIRECTION ( 'NONE',  ( -0.000000000000000000, 0.000000000000000000, -1.000000000000000000 ) ) ;
#8257=CARTESIAN_POINT ( 'NONE',  ( 0.000000000000000000, 0.000000000000000000, 65.00000000000000000 ) ) ;
#8295=DIRECTION ( 'NONE',  ( 0.000000000000000000, 0.000000000000000000, -1.000000000000000000 ) ) ;
#8299=CARTESIAN_POINT ( 'NONE',  ( -3.799999999999999822, 4.653657836759942730E-16, -44.50000000000000000 ) ) ;
#8321=EDGE_CURVE ( 'NONE', #31925, #29341, #30291, .T. ) ;
#8328=DIRECTION ( 'NONE',  ( 0.000000000000000000, 0.000000000000000000, -1.000000000000000000 ) ) ;
#8350=DIRECTION ( 'NONE',  ( 0.000000000000000000, 0.000000000000000000, 1.000000000000000000 ) ) ;
#8364=EDGE_CURVE ( 'NONE', #17651, #15054, #34577, .T. ) ;
#8369=PLANE ( 'NONE',  #3965 ) ;
#8370=CARTESIAN_POINT ( 'NONE',  ( 0.000000000000000000, 0.000000000000000000, 60.00000000000000000 ) ) ;
#8374=DIRECTION ( 'NONE',  ( -0.000000000000000000, 0.000000000000000000, -1.000000000000000000 ) ) ;
#8390=LINE ( 'NONE', #3373, #34819 ) ;
#8391=ADVANCED_FACE ( 'NONE', ( #4531 ), #12965, .T. ) ;
#8410=CIRCLE ( 'NONE', #29145, 3.799999999999999822 ) ;
#8411=EDGE_CURVE ( 'NONE', #16728, #9474, #29788, .T. ) ;
#8415=CIRCLE ( 'NONE', #3840, 4.000000000000000000 ) ;
#8418=ORIENTED_EDGE ( 'NONE', *, *, #9445, .F. ) ;
#8463=CARTESIAN_POINT ( 'NONE',  ( 3.799999999999999822, 0.000000000000000000, 60.00000000000000000 ) ) ;
#8479=CYLINDRICAL_SURFACE ( 'NONE', #16605, 4.000000000000000000 ) ;
#8517=EDGE_CURVE ( 'NONE', #17838, #7584, #10446, .T. ) ;
#8552=CYLINDRICAL_SURFACE ( 'NONE', #7025, 3.799999999999999822 ) ;
#8560=DIRECTION ( 'NONE',  ( -1.000000000000000000, 0.000000000000000000, 0.000000000000000000 ) ) ;
#8568=DIRECTION ( 'NONE',  ( 0.000000000000000000, 0.000000000000000000, -1.000000000000000000 ) ) ;
#8591=EDGE_CURVE ( 'NONE', #34626, #28884, #379, .T. ) ;
#8675=VERTEX_POINT ( 'NONE', #8777 ) ;
#8691=VECTOR ( 'NONE', #18340, 1000.000000000000000 ) ;
#8739=ORIENTED_EDGE ( 'NONE', *, *, #31053, .T. ) ;
#8743=CARTESIAN_POINT ( 'NONE',  ( -4.000000000000000000, 0.000000000000000000, -55.00000000000000000 ) ) ;
#8777=CARTESIAN_POINT ( 'NONE',  ( -4.000000000000000000, 0.000000000000000000, 36.00000000000000000 ) ) ;
#8811=CIRCLE ( 'NONE', #28952, 3.799999999999999822 ) ;
#8817=FACE_BOUND ( 'NONE', #12432, .T. ) ;
#8821=EDGE_CURVE ( 'NONE', #33549, #28885, #27999, .T. ) ;
#8911=VECTOR ( 'NONE', #28200, 1000.000000000000000 ) ;
#8922=CARTESIAN_POINT ( 'NONE',  ( 0.000000000000000000, 0.000000000000000000, -31.10000000000000142 ) ) ;
#8932=CARTESIAN_POINT ( 'NONE',  ( 4.000000000000000000, 4.898587196589412829E-16, -65.00000000000000000 ) ) ;
#8937=CARTESIAN_POINT ( 'NONE',  ( 0.000000000000000000, 0.000000000000000000, -32.00000000000000000 ) ) ;
#8976=VERTEX_POINT ( 'NONE', #28948 ) ;
#8989=CIRCLE ( 'NONE', #13608, 4.000000000000000000 ) ;
#9014=CARTESIAN_POINT ( 'NONE',  ( 0.000000000000000000, 0.000000000000000000, -40.89999999999999858 ) ) ;
#9036=ADVANCED_FACE ( 'NONE', ( #23907 ), #10223, .T. ) ;
#9074=DIRECTION ( 'NONE',  ( -1.000000000000000000, 0.000000000000000000, 0.000000000000000000 ) ) ;
#9083=ADVANCED_FACE ( 'NONE', ( #8041 ), #5528, .T. ) ;
#9098=CYLINDRICAL_SURFACE ( 'NONE', #18554, 3.799999999999999822 ) ;
#9131=AXIS2_PLACEMENT_3D ( 'NONE', #35367, #32469, #2792 ) ;
#9145=DIRECTION ( 'NONE',  ( -0.000000000000000000, 0.000000000000000000, -1.000000000000000000 ) ) ;
#9190=DIRECTION ( 'NONE',  ( 0.000000000000000000, 1.000000000000000000, 0.000000000000000000 ) ) ;
#9209=ORIENTED_EDGE ( 'NONE', *, *, #33270, .T. ) ;
#9216=DIRECTION ( 'NONE',  ( 0.000000000000000000, 0.000000000000000000, -1.000000000000000000 ) ) ;
#9233=DIRECTION ( 'NONE',  ( -1.000000000000000000, 0.000000000000000000, 0.000000000000000000 ) ) ;
#9244=ORIENTED_EDGE ( 'NONE', *, *, #33270, .F. ) ;
#9256=ORIENTED_EDGE ( 'NONE', *, *, #1089, .F. ) ;
#9289=VERTEX_POINT ( 'NONE', #21317 ) ;
#9298=PRESENTATION_STYLE_ASSIGNMENT (( #15208 ) ) ;
#9306=DIRECTION ( 'NONE',  ( 1.000000000000000000, 0.000000000000000000, 0.000000000000000000 ) ) ;
#9316=CIRCLE ( 'NONE', #24848, 4.000000000000000000 ) ;
#9338=CARTESIAN_POINT ( 'NONE',  ( -4.000000000000000000, 0.000000000000000000, 35.10000000000000142 ) ) ;
#9368=CARTESIAN_POINT ( 'NONE',  ( 4.000000000000000000, 4.898587196589412829E-16, 65.00000000000000000 ) ) ;
#9445=EDGE_CURVE ( 'NONE', #19012, #7584, #3900, .T. ) ;
#9465=DIRECTION ( 'NONE',  ( 0.000000000000000000, 0.000000000000000000, -1.000000000000000000 ) ) ;
#9474=VERTEX_POINT ( 'NONE', #2274 ) ;
#9483=VERTEX_POINT ( 'NONE', #17504 ) ;
#9499=FACE_OUTER_BOUND ( 'NONE', #31702, .T. ) ;
#9517=CIRCLE ( 'NONE', #22174, 3.799999999999999822 ) ;
#9523=CARTESIAN_POINT ( 'NONE',  ( 0.000000000000000000, 0.000000000000000000, -31.10000000000000142 ) ) ;
#9545=DIRECTION ( 'NONE',  ( 0.000000000000000000, 0.000000000000000000, 1.000000000000000000 ) ) ;
#9548=ORIENTED_EDGE ( 'NONE', *, *, #8321, .F. ) ;
#9561=FACE_BOUND ( 'NONE', #12157, .T. ) ;
#9601=CIRCLE ( 'NONE', #14193, 3.799999999999999822 ) ;
#9613=ORIENTED_EDGE ( 'NONE', *, *, #1551, .T. ) ;
#9647=ORIENTED_EDGE ( 'NONE', *, *, #3659, .T. ) ;
#9671=DIRECTION ( 'NONE',  ( 1.110223024625156540E-16, 1.000000000000000000, 0.000000000000000000 ) ) ;
#9688=DIRECTION ( 'NONE',  ( 0.000000000000000000, 0.000000000000000000, 1.000000000000000000 ) ) ;
#9708=DIRECTION ( 'NONE',  ( 0.000000000000000000, 0.000000000000000000, -1.000000000000000000 ) ) ;
#9739=EDGE_CURVE ( 'NONE', #15935, #22572, #21711, .T. ) ;
#9778=DIRECTION ( 'NONE',  ( -1.000000000000000000, 0.000000000000000000, 0.000000000000000000 ) ) ;
#9825=SURFACE_STYLE_FILL_AREA ( #26401 ) ;
#9884=FACE_OUTER_BOUND ( 'NONE', #23105, .T. ) ;
#9897=CARTESIAN_POINT ( 'NONE',  ( 0.000000000000000000, 0.000000000000000000, -55.00000000000000000 ) ) ;
#9901=EDGE_CURVE ( 'NONE', #22572, #1546, #10488, .T. ) ;
#9933=EDGE_LOOP ( 'NONE', ( #27048, #4645 ) ) ;
#9975=CARTESIAN_POINT ( 'NONE',  ( 3.799999999999999822, 0.000000000000000000, 36.00000000000000000 ) ) ;
#9978=EDGE_CURVE ( 'NONE', #17384, #33209, #25859, .T. ) ;
#9981=AXIS2_PLACEMENT_3D ( 'NONE', #3753, #22996, #25542 ) ;
#10039=CARTESIAN_POINT ( 'NONE',  ( 0.000000000000000000, 0.000000000000000000, 60.90000000000001279 ) ) ;
#10066=VERTEX_POINT ( 'NONE', #33868 ) ;
#10076=CARTESIAN_POINT ( 'NONE',  ( 0.000000000000000000, 0.000000000000000000, 36.00000000000000000 ) ) ;
#10129=CARTESIAN_POINT ( 'NONE',  ( -3.799999999999999822, 4.653657836759942730E-16, -31.10000000000000142 ) ) ;
#10141=DIRECTION ( 'NONE',  ( 0.000000000000000000, 0.000000000000000000, -1.000000000000000000 ) ) ;
#10157=DIRECTION ( 'NONE',  ( 1.000000000000000000, 0.000000000000000000, 0.000000000000000000 ) ) ;
#10182=CARTESIAN_POINT ( 'NONE',  ( -3.799999999999999822, 4.653657836759942730E-16, -53.39999999999999858 ) ) ;
#10209=CARTESIAN_POINT ( 'NONE',  ( 0.000000000000000000, 0.000000000000000000, -40.89999999999999858 ) ) ;
#10223=CYLINDRICAL_SURFACE ( 'NONE', #19943, 3.799999999999999822 ) ;
#10226=CYLINDRICAL_SURFACE ( 'NONE', #22431, 3.799999999999999822 ) ;
#10243=ORIENTED_EDGE ( 'NONE', *, *, #31569, .T. ) ;
#10244=EDGE_LOOP ( 'NONE', ( #25621, #23956, #33085, #14672 ) ) ;
#10291=CARTESIAN_POINT ( 'NONE',  ( 0.000000000000000000, 0.000000000000000000, 65.00000000000000000 ) ) ;
#10296=( NAMED_UNIT ( * ) PLANE_ANGLE_UNIT ( ) SI_UNIT ( $, .RADIAN. ) );
#10326=CARTESIAN_POINT ( 'NONE',  ( 0.000000000000000000, 0.000000000000000000, -44.50000000000000000 ) ) ;
#10329=DIRECTION ( 'NONE',  ( 0.000000000000000000, 0.000000000000000000, -1.000000000000000000 ) ) ;
#10332=EDGE_LOOP ( 'NONE', ( #20354, #3125, #15214, #22173 ) ) ;
#10366=DIRECTION ( 'NONE',  ( 1.110223024625156540E-16, 1.000000000000000000, 0.000000000000000000 ) ) ;
#10375=DIRECTION ( 'NONE',  ( -1.000000000000000000, 0.000000000000000000, 0.000000000000000000 ) ) ;
#10382=ADVANCED_FACE ( 'NONE', ( #33960, #34137 ), #17018, .T. ) ;
#10430=EDGE_LOOP ( 'NONE', ( #2738, #25566 ) ) ;
#10446=LINE ( 'NONE', #21406, #27969 ) ;
#10461=CARTESIAN_POINT ( 'NONE',  ( -4.000000000000000000, 0.000000000000000000, 65.00000000000000000 ) ) ;
#10463=COLOUR_RGB ( '', 0.66274510, 0.83137255, 0.94901961) ;
#10481=DIRECTION ( 'NONE',  ( -0.000000000000000000, 0.000000000000000000, -1.000000000000000000 ) ) ;
#10488=LINE ( 'NONE', #8299, #33803 ) ;
#10530=CARTESIAN_POINT ( 'NONE',  ( 3.799999999999999822, 0.000000000000000000, -52.50000000000000000 ) ) ;
#10539=VERTEX_POINT ( 'NONE', #11802 ) ;
#10553=CARTESIAN_POINT ( 'NONE',  ( 0.000000000000000000, 0.000000000000000000, 55.00000000000000711 ) ) ;
#10558=EDGE_LOOP ( 'NONE', ( #19768, #31078 ) ) ;
#10576=FACE_OUTER_BOUND ( 'NONE', #12540, .T. ) ;
#10629=EDGE_LOOP ( 'NONE', ( #30452, #32949, #34307, #569 ) ) ;
#10635=EDGE_LOOP ( 'NONE', ( #27706, #33507 ) ) ;
#10642=ADVANCED_FACE ( 'NONE', ( #20961 ), #1726, .T. ) ;
#10655=AXIS2_PLACEMENT_3D ( 'NONE', #8257, #8083, #158 ) ;
#10669=CARTESIAN_POINT ( 'NONE',  ( 3.799999999999999822, 0.000000000000000000, 35.10000000000000142 ) ) ;
#10673=ORIENTED_EDGE ( 'NONE', *, *, #16872, .F. ) ;
#10678=EDGE_CURVE ( 'NONE', #28884, #34626, #28217, .T. ) ;
#10690=VERTEX_POINT ( 'NONE', #19160 ) ;
#10701=AXIS2_PLACEMENT_3D ( 'NONE', #4389, #7777, #9778 ) ;
#10708=CIRCLE ( 'NONE', #19325, 3.799999999999999822 ) ;
#10730=EDGE_LOOP ( 'NONE', ( #9256, #4729, #21645, #18333 ) ) ;
#10734=EDGE_CURVE ( 'NONE', #891, #16728, #27110, .T. ) ;
#10794=LINE ( 'NONE', #2528, #17133 ) ;
#10802=CARTESIAN_POINT ( 'NONE',  ( 0.000000000000000000, 0.000000000000000000, -32.00000000000000000 ) ) ;
#10808=EDGE_LOOP ( 'NONE', ( #32725, #19504, #19347, #18865, #7430 ) ) ;
#10817=FACE_OUTER_BOUND ( 'NONE', #20873, .T. ) ;
#10879=PLANE ( 'NONE',  #22562 ) ;
#10901=DIRECTION ( 'NONE',  ( -1.000000000000000000, 0.000000000000000000, 0.000000000000000000 ) ) ;
#10916=ORIENTED_EDGE ( 'NONE', *, *, #34140, .T. ) ;
#10950=AXIS2_PLACEMENT_3D ( 'NONE', #4440, #24933, #10901 ) ;
#10952=CIRCLE ( 'NONE', #602, 3.799999999999999822 ) ;
#10968=EDGE_CURVE ( 'NONE', #29341, #32249, #6718, .T. ) ;
#10975=CARTESIAN_POINT ( 'NONE',  ( 3.799999999999999822, 0.000000000000000000, -31.10000000000000142 ) ) ;
#11045=EDGE_LOOP ( 'NONE', ( #16751, #11341, #49, #15005 ) ) ;
#11065=DIRECTION ( 'NONE',  ( 0.000000000000000000, 0.000000000000000000, -1.000000000000000000 ) ) ;
#11069=EDGE_CURVE ( 'NONE', #17029, #17838, #45, .T. ) ;
#11083=CARTESIAN_POINT ( 'NONE',  ( 5.400000000000071410, 0.9999999999999662492, 45.00000000000000711 ) ) ;
#11160=CARTESIAN_POINT ( 'NONE',  ( 0.000000000000000000, 0.000000000000000000, -32.00000000000000000 ) ) ;
#11284=EDGE_LOOP ( 'NONE', ( #27058, #22049, #25258, #24373 ) ) ;
#11301=AXIS2_PLACEMENT_3D ( 'NONE', #19539, #14148, #2847 ) ;
#11305=AXIS2_PLACEMENT_3D ( 'NONE', #15304, #11912, #7036 ) ;
#11308=VECTOR ( 'NONE', #1949, 1000.000000000000000 ) ;
#11309=VERTEX_POINT ( 'NONE', #21995 ) ;
#11323=VECTOR ( 'NONE', #13252, 1000.000000000000000 ) ;
#11327=AXIS2_PLACEMENT_3D ( 'NONE', #17514, #23471, #26170 ) ;
#11335=COLOUR_RGB ( '', 0.66274510, 0.83137255, 0.94901961) ;
#11341=ORIENTED_EDGE ( 'NONE', *, *, #31891, .T. ) ;
#11355=ORIENTED_EDGE ( 'NONE', *, *, #31244, .T. ) ;
#11483=FACE_OUTER_BOUND ( 'NONE', #26806, .T. ) ;
#11510=LINE ( 'NONE', #3771, #18856 ) ;
#11520=ADVANCED_FACE ( 'NONE', ( #20699, #9561 ), #6675, .T. ) ;
#11549=DIRECTION ( 'NONE',  ( -1.000000000000000000, 0.000000000000000000, 0.000000000000000000 ) ) ;
#11581=DIRECTION ( 'NONE',  ( -1.000000000000000000, 0.000000000000000000, 0.000000000000000000 ) ) ;
#11603=ORIENTED_EDGE ( 'NONE', *, *, #6419, .T. ) ;
#11638=AXIS2_PLACEMENT_3D ( 'NONE', #35161, #10481, #35512 ) ;
#11649=VERTEX_POINT ( 'NONE', #33813 ) ;
#11708=FACE_BOUND ( 'NONE', #34433, .T. ) ;
#11712=DIRECTION ( 'NONE',  ( -1.000000000000000000, 0.000000000000000000, 0.000000000000000000 ) ) ;
#11715=CARTESIAN_POINT ( 'NONE',  ( 0.000000000000000000, 0.000000000000000000, -43.60000000000000142 ) ) ;
#11729=EDGE_LOOP ( 'NONE', ( #30868, #32259, #17540, #31830 ) ) ;
#11758=CARTESIAN_POINT ( 'NONE',  ( 0.000000000000000000, 0.000000000000000000, -55.89999999999999858 ) ) ;
#11790=AXIS2_PLACEMENT_3D ( 'NONE', #10039, #29316, #32185 ) ;
#11795=AXIS2_PLACEMENT_3D ( 'NONE', #16809, #17513, #3507 ) ;
#11802=CARTESIAN_POINT ( 'NONE',  ( 3.872983346207489852, 0.9999999999999522604, -44.50000000000000000 ) ) ;
#11805=LINE ( 'NONE', #28208, #19824 ) ;
#11856=DIRECTION ( 'NONE',  ( -1.000000000000000000, 0.000000000000000000, 0.000000000000000000 ) ) ;
#11857=CARTESIAN_POINT ( 'NONE',  ( -4.000000000000000000, 0.000000000000000000, 60.00000000000000000 ) ) ;
#11864=CARTESIAN_POINT ( 'NONE',  ( 0.000000000000000000, 0.000000000000000000, 55.00000000000000711 ) ) ;
#11888=DIRECTION ( 'NONE',  ( -1.000000000000000000, 0.000000000000000000, 0.000000000000000000 ) ) ;
#11912=DIRECTION ( 'NONE',  ( 0.000000000000000000, 0.000000000000000000, -1.000000000000000000 ) ) ;
#11914=ORIENTED_EDGE ( 'NONE', *, *, #5616, .T. ) ;
#11922=ORIENTED_EDGE ( 'NONE', *, *, #1708, .F. ) ;
#11938=CIRCLE ( 'NONE', #18279, 4.000000000000000000 ) ;
#11953=DIRECTION ( 'NONE',  ( -0.000000000000000000, 0.000000000000000000, -1.000000000000000000 ) ) ;
#11955=DIRECTION ( 'NONE',  ( 1.000000000000000000, 0.000000000000000000, 0.000000000000000000 ) ) ;
#11992=VECTOR ( 'NONE', #23521, 1000.000000000000000 ) ;
#12037=ORIENTED_EDGE ( 'NONE', *, *, #34873, .T. ) ;
#12076=EDGE_LOOP ( 'NONE', ( #12777, #4920, #2215, #18524 ) ) ;
#12103=ADVANCED_FACE ( 'NONE', ( #33807 ), #32969, .F. ) ;
#12106=CARTESIAN_POINT ( 'NONE',  ( 1.110223024625156540E-13, -1.000000000000042633, -44.50000000000000000 ) ) ;
#12122=CYLINDRICAL_SURFACE ( 'NONE', #161, 3.799999999999999822 ) ;
#12147=AXIS2_PLACEMENT_3D ( 'NONE', #31663, #22847, #1250 ) ;
#12157=EDGE_LOOP ( 'NONE', ( #18346, #2513 ) ) ;
#12178=DIRECTION ( 'NONE',  ( 1.000000000000000000, -1.110223024625156540E-16, 0.000000000000000000 ) ) ;
#12249=CARTESIAN_POINT ( 'NONE',  ( 0.000000000000000000, 0.000000000000000000, 65.00000000000000000 ) ) ;
#12350=ORIENTED_EDGE ( 'NONE', *, *, #34791, .F. ) ;
#12432=EDGE_LOOP ( 'NONE', ( #53, #23773 ) ) ;
#12450=CARTESIAN_POINT ( 'NONE',  ( 0.000000000000000000, 0.000000000000000000, 65.00000000000000000 ) ) ;
#12478=DIRECTION ( 'NONE',  ( 0.000000000000000000, 0.000000000000000000, -1.000000000000000000 ) ) ;
#12493=CARTESIAN_POINT ( 'NONE',  ( 9.714451465470119729E-14, 0.9999999999999870104, 45.00000000000000711 ) ) ;
#12494=ORIENTED_EDGE ( 'NONE', *, *, #27762, .T. ) ;
#12533=CIRCLE ( 'NONE', #30355, 4.000000000000000000 ) ;
#12534=DIRECTION ( 'NONE',  ( -1.000000000000000000, 0.000000000000000000, 0.000000000000000000 ) ) ;
#12540=EDGE_LOOP ( 'NONE', ( #14344, #445, #6103, #33565 ) ) ;
#12548=CARTESIAN_POINT ( 'NONE',  ( 4.000000000000000000, 4.898587196589412829E-16, 65.00000000000000000 ) ) ;
#12568=VECTOR ( 'NONE', #30557, 1000.000000000000000 ) ;
#12580=ORIENTED_EDGE ( 'NONE', *, *, #16775, .F. ) ;
#12582=DIRECTION ( 'NONE',  ( 1.110223024625156540E-16, 1.000000000000000000, 0.000000000000000000 ) ) ;
#12588=AXIS2_PLACEMENT_3D ( 'NONE', #20590, #31938, #10157 ) ;
#12603=CARTESIAN_POINT ( 'NONE',  ( 0.000000000000000000, 0.000000000000000000, -53.39999999999999858 ) ) ;
#12617=ORIENTED_EDGE ( 'NONE', *, *, #24673, .T. ) ;
#12683=VERTEX_POINT ( 'NONE', #7906 ) ;
#12688=LINE ( 'NONE', #20761, #28681 ) ;
#12699=VERTEX_POINT ( 'NONE', #10975 ) ;
#12709=CARTESIAN_POINT ( 'NONE',  ( 9.714451465470119729E-14, 0.9999999999999870104, -32.00000000000000000 ) ) ;
#12710=ORIENTED_EDGE ( 'NONE', *, *, #20745, .T. ) ;
#12725=DIRECTION ( 'NONE',  ( 0.000000000000000000, 0.000000000000000000, 1.000000000000000000 ) ) ;
#12762=ORIENTED_EDGE ( 'NONE', *, *, #6614, .F. ) ;
#12772=EDGE_LOOP ( 'NONE', ( #30269, #14176, #25739, #35452 ) ) ;
#12776=DIRECTION ( 'NONE',  ( 0.000000000000000000, 0.000000000000000000, -1.000000000000000000 ) ) ;
#12777=ORIENTED_EDGE ( 'NONE', *, *, #8517, .F. ) ;
#12790=ORIENTED_EDGE ( 'NONE', *, *, #16113, .F. ) ;
#12793=EDGE_LOOP ( 'NONE', ( #27218, #17105, #11603, #9209 ) ) ;
#12808=EDGE_CURVE ( 'NONE', #19295, #11649, #27043, .T. ) ;
#12833=FACE_OUTER_BOUND ( 'NONE', #11045, .T. ) ;
#12854=CARTESIAN_POINT ( 'NONE',  ( 5.400000000000085620, -1.000000000000049516, 55.00000000000000711 ) ) ;
#12873=EDGE_CURVE ( 'NONE', #24508, #5329, #33821, .T. ) ;
#12898=AXIS2_PLACEMENT_3D ( 'NONE', #34953, #26664, #35129 ) ;
#12915=DIRECTION ( 'NONE',  ( -1.000000000000000000, 0.000000000000000000, 0.000000000000000000 ) ) ;
#12922=DIRECTION ( 'NONE',  ( 0.000000000000000000, 0.000000000000000000, 1.000000000000000000 ) ) ;
#12947=CARTESIAN_POINT ( 'NONE',  ( 4.000000000000000000, 4.898587196589412829E-16, 65.00000000000000000 ) ) ;
#12965=CYLINDRICAL_SURFACE ( 'NONE', #15378, 3.799999999999999822 ) ;
#12988=ORIENTED_EDGE ( 'NONE', *, *, #6154, .F. ) ;
#13024=FACE_OUTER_BOUND ( 'NONE', #18835, .T. ) ;
#13029=DIRECTION ( 'NONE',  ( -1.000000000000000000, 0.000000000000000000, 0.000000000000000000 ) ) ;
#13120=FACE_OUTER_BOUND ( 'NONE', #22525, .T. ) ;
#13141=ORIENTED_EDGE ( 'NONE', *, *, #29590, .F. ) ;
#13169=ORIENTED_EDGE ( 'NONE', *, *, #9901, .F. ) ;
#13199=ORIENTED_EDGE ( 'NONE', *, *, #63, .F. ) ;
#13203=ADVANCED_FACE ( 'NONE', ( #4663 ), #10226, .T. ) ;
#13233=LINE ( 'NONE', #16430, #13630 ) ;
#13252=DIRECTION ( 'NONE',  ( 0.000000000000000000, 0.000000000000000000, 1.000000000000000000 ) ) ;
#13300=ORIENTED_EDGE ( 'NONE', *, *, #21511, .F. ) ;
#13305=ADVANCED_FACE ( 'NONE', ( #21527 ), #5873, .T. ) ;
#13348=DIRECTION ( 'NONE',  ( -0.000000000000000000, 0.000000000000000000, -1.000000000000000000 ) ) ;
#13375=ADVANCED_BREP_SHAPE_REPRESENTATION ( '', ( #34226, #21307 ), #26556 ) ;
#13395=FACE_OUTER_BOUND ( 'NONE', #28516, .T. ) ;
#13408=FACE_BOUND ( 'NONE', #10430, .T. ) ;
#13409=ORIENTED_EDGE ( 'NONE', *, *, #10734, .T. ) ;
#13424=VERTEX_POINT ( 'NONE', #22419 ) ;
#13455=CARTESIAN_POINT ( 'NONE',  ( 0.000000000000000000, 0.000000000000000000, 65.00000000000000000 ) ) ;
#13475=LINE ( 'NONE', #5383, #32664 ) ;
#13482=AXIS2_PLACEMENT_3D ( 'NONE', #4312, #12582, #1604 ) ;
#13512=CIRCLE ( 'NONE', #22678, 4.000000000000000000 ) ;
#13526=CIRCLE ( 'NONE', #34209, 3.799999999999999822 ) ;
#13530=ADVANCED_FACE ( 'NONE', ( #28906, #15027 ), #18082, .F. ) ;
#13540=DIRECTION ( 'NONE',  ( 0.000000000000000000, 0.000000000000000000, -1.000000000000000000 ) ) ;
#13545=DIRECTION ( 'NONE',  ( 0.000000000000000000, 0.000000000000000000, 1.000000000000000000 ) ) ;
#13562=CIRCLE ( 'NONE', #2656, 3.799999999999999822 ) ;
#13608=AXIS2_PLACEMENT_3D ( 'NONE', #11715, #31345, #11549 ) ;
#13630=VECTOR ( 'NONE', #24042, 1000.000000000000000 ) ;
#13633=ORIENTED_EDGE ( 'NONE', *, *, #29094, .T. ) ;
#13640=DIRECTION ( 'NONE',  ( -0.000000000000000000, 0.000000000000000000, -1.000000000000000000 ) ) ;
#13646=LINE ( 'NONE', #5205, #27290 ) ;
#13668=AXIS2_PLACEMENT_3D ( 'NONE', #10291, #13348, #15837 ) ;
#13676=CIRCLE ( 'NONE', #19394, 3.799999999999999822 ) ;
#13711=CARTESIAN_POINT ( 'NONE',  ( 0.000000000000000000, 0.000000000000000000, 45.00000000000000711 ) ) ;
#13729=CARTESIAN_POINT ( 'NONE',  ( 1.110223024625156540E-13, -1.000000000000042633, -32.00000000000000000 ) ) ;
#13785=EDGE_LOOP ( 'NONE', ( #16563, #20119, #9613, #12494 ) ) ;
#13791=FACE_OUTER_BOUND ( 'NONE', #10332, .T. ) ;
#13815=CARTESIAN_POINT ( 'NONE',  ( 1.110223024625156540E-13, -1.000000000000042633, 53.00000000000000711 ) ) ;
#13859=EDGE_LOOP ( 'NONE', ( #22435, #3643, #184, #33805 ) ) ;
#14000=EDGE_CURVE ( 'NONE', #11309, #32739, #2674, .T. ) ;
#14010=EDGE_CURVE ( 'NONE', #7515, #31797, #24628, .T. ) ;
#14030=CIRCLE ( 'NONE', #2576, 4.000000000000000000 ) ;
#14039=ADVANCED_FACE ( 'NONE', ( #30552 ), #3196, .F. ) ;
#14040=ADVANCED_FACE ( 'NONE', ( #33789 ), #30387, .F. ) ;
#14055=VERTEX_POINT ( 'NONE', #8743 ) ;
#14086=CARTESIAN_POINT ( 'NONE',  ( 3.872983346207517386, -1.000000000000028644, -44.50000000000000000 ) ) ;
#14148=DIRECTION ( 'NONE',  ( 0.000000000000000000, 0.000000000000000000, -1.000000000000000000 ) ) ;
#14157=VERTEX_POINT ( 'NONE', #28742 ) ;
#14176=ORIENTED_EDGE ( 'NONE', *, *, #23119, .T. ) ;
#14193=AXIS2_PLACEMENT_3D ( 'NONE', #10326, #32108, #13029 ) ;
#14206=PLANE ( 'NONE',  #1057 ) ;
#14284=EDGE_CURVE ( 'NONE', #7515, #9483, #27954, .T. ) ;
#14296=EDGE_CURVE ( 'NONE', #28885, #5282, #15037, .T. ) ;
#14301=ORIENTED_EDGE ( 'NONE', *, *, #6614, .T. ) ;
#14341=EDGE_CURVE ( 'NONE', #21809, #1825, #29633, .T. ) ;
#14344=ORIENTED_EDGE ( 'NONE', *, *, #14688, .F. ) ;
#14384=AXIS2_PLACEMENT_3D ( 'NONE', #21479, #29966, #30138 ) ;
#14405=PLANE ( 'NONE',  #14588 ) ;
#14429=ORIENTED_EDGE ( 'NONE', *, *, #29628, .T. ) ;
#14433=ORIENTED_EDGE ( 'NONE', *, *, #4845, .T. ) ;
#14480=CYLINDRICAL_SURFACE ( 'NONE', #21993, 4.000000000000000000 ) ;
#14527=DIRECTION ( 'NONE',  ( -1.000000000000000000, 0.000000000000000000, 0.000000000000000000 ) ) ;
#14530=LINE ( 'NONE', #17589, #30256 ) ;
#14535=FACE_OUTER_BOUND ( 'NONE', #23524, .T. ) ;
#14588=AXIS2_PLACEMENT_3D ( 'NONE', #17280, #32674, #19971 ) ;
#14627=LINE ( 'NONE', #25637, #17977 ) ;
#14632=DIRECTION ( 'NONE',  ( 0.000000000000000000, 0.000000000000000000, -1.000000000000000000 ) ) ;
#14636=CARTESIAN_POINT ( 'NONE',  ( -3.799999999999999822, 4.653657836759942730E-16, -40.00000000000000000 ) ) ;
#14672=ORIENTED_EDGE ( 'NONE', *, *, #2901, .F. ) ;
#14678=ORIENTED_EDGE ( 'NONE', *, *, #29590, .T. ) ;
#14688=EDGE_CURVE ( 'NONE', #5174, #891, #18207, .T. ) ;
#14748=DIRECTION ( 'NONE',  ( 0.000000000000000000, 0.000000000000000000, -1.000000000000000000 ) ) ;
#14763=PLANE ( 'NONE',  #24970 ) ;
#14791=ADVANCED_FACE ( 'NONE', ( #4050 ), #31744, .T. ) ;
#14818=DIRECTION ( 'NONE',  ( -0.000000000000000000, 0.000000000000000000, -1.000000000000000000 ) ) ;
#14821=DIRECTION ( 'NONE',  ( 0.000000000000000000, 0.000000000000000000, 1.000000000000000000 ) ) ;
#14825=EDGE_CURVE ( 'NONE', #22572, #15935, #9601, .T. ) ;
#14843=DIRECTION ( 'NONE',  ( -1.000000000000000000, 0.000000000000000000, 0.000000000000000000 ) ) ;
#14859=CARTESIAN_POINT ( 'NONE',  ( 4.000000000000000000, 4.898587196589412829E-16, 36.00000000000000000 ) ) ;
#14869=ORIENTED_EDGE ( 'NONE', *, *, #10678, .F. ) ;
#14882=VERTEX_POINT ( 'NONE', #32285 ) ;
#14960=EDGE_CURVE ( 'NONE', #21576, #28168, #31448, .T. ) ;
#14990=DIRECTION ( 'NONE',  ( 0.000000000000000000, 0.000000000000000000, 1.000000000000000000 ) ) ;
#15000=VERTEX_POINT ( 'NONE', #27940 ) ;
#15004=ORIENTED_EDGE ( 'NONE', *, *, #26373, .F. ) ;
#15005=ORIENTED_EDGE ( 'NONE', *, *, #6968, .F. ) ;
#15027=FACE_BOUND ( 'NONE', #6646, .T. ) ;
#15037=LINE ( 'NONE', #33965, #23436 ) ;
#15054=VERTEX_POINT ( 'NONE', #16935 ) ;
#15077=FACE_OUTER_BOUND ( 'NONE', #7027, .T. ) ;
#15083=DIRECTION ( 'NONE',  ( 1.000000000000000000, 0.000000000000000000, 0.000000000000000000 ) ) ;
#15109=DIRECTION ( 'NONE',  ( -1.000000000000000000, 0.000000000000000000, 0.000000000000000000 ) ) ;
#15128=ORIENTED_EDGE ( 'NONE', *, *, #33644, .F. ) ;
#15144=CIRCLE ( 'NONE', #2547, 4.000000000000000000 ) ;
#15198=CARTESIAN_POINT ( 'NONE',  ( 3.799999999999999822, 0.000000000000000000, -40.00000000000000000 ) ) ;
#15201=ADVANCED_FACE ( 'NONE', ( #1290 ), #31000, .T. ) ;
#15208=SURFACE_STYLE_USAGE ( .BOTH. , #18284 ) ;
#15214=ORIENTED_EDGE ( 'NONE', *, *, #34592, .T. ) ;
#15242=DIRECTION ( 'NONE',  ( 1.000000000000000000, -1.110223024625156540E-16, 0.000000000000000000 ) ) ;
#15266=LINE ( 'NONE', #23568, #17890 ) ;
#15279=DIRECTION ( 'NONE',  ( 0.000000000000000000, 0.000000000000000000, 1.000000000000000000 ) ) ;
#15304=CARTESIAN_POINT ( 'NONE',  ( 0.000000000000000000, 0.000000000000000000, -55.00000000000000000 ) ) ;
#15328=CARTESIAN_POINT ( 'NONE',  ( 0.000000000000000000, 0.000000000000000000, 65.00000000000000000 ) ) ;
#15351=EDGE_LOOP ( 'NONE', ( #18267, #31303, #19129, #26634 ) ) ;
#15358=DIRECTION ( 'NONE',  ( -0.000000000000000000, 0.000000000000000000, -1.000000000000000000 ) ) ;
#15378=AXIS2_PLACEMENT_3D ( 'NONE', #28988, #27011, #34754 ) ;
#15396=ORIENTED_EDGE ( 'NONE', *, *, #17238, .F. ) ;
#15427=ORIENTED_EDGE ( 'NONE', *, *, #28355, .F. ) ;
#15456=DIRECTION ( 'NONE',  ( -1.000000000000000000, 0.000000000000000000, 0.000000000000000000 ) ) ;
#15486=ORIENTED_EDGE ( 'NONE', *, *, #5738, .T. ) ;
#15491=DIRECTION ( 'NONE',  ( -1.000000000000000000, 0.000000000000000000, 0.000000000000000000 ) ) ;
#15508=CARTESIAN_POINT ( 'NONE',  ( 4.000000000000000000, 4.898587196589412829E-16, -53.39999999999999858 ) ) ;
#15509=VERTEX_POINT ( 'NONE', #8463 ) ;
#15530=FACE_OUTER_BOUND ( 'NONE', #28077, .T. ) ;
#15667=FILL_AREA_STYLE_COLOUR ( '', #10463 ) ;
#15713=CARTESIAN_POINT ( 'NONE',  ( 1.110223024625156540E-13, -1.000000000000042633, -32.00000000000000000 ) ) ;
#15759=CARTESIAN_POINT ( 'NONE',  ( -3.799999999999999822, 4.653657836759942730E-16, -53.39999999999999858 ) ) ;
#15789=CIRCLE ( 'NONE', #10655, 4.000000000000000000 ) ;
#15823=EDGE_CURVE ( 'NONE', #28885, #23250, #13475, .T. ) ;
#15837=DIRECTION ( 'NONE',  ( -1.000000000000000000, 0.000000000000000000, 0.000000000000000000 ) ) ;
#15877=CARTESIAN_POINT ( 'NONE',  ( 0.000000000000000000, 0.000000000000000000, -40.00000000000000711 ) ) ;
#15935=VERTEX_POINT ( 'NONE', #27697 ) ;
#15944=DIRECTION ( 'NONE',  ( -1.000000000000000000, 0.000000000000000000, 0.000000000000000000 ) ) ;
#15961=CARTESIAN_POINT ( 'NONE',  ( 5.400000000000071410, 0.9999999999999662492, 53.00000000000000711 ) ) ;
#15997=CARTESIAN_POINT ( 'NONE',  ( 5.400000000000085620, -1.000000000000049516, 53.00000000000000711 ) ) ;
#16012=DIRECTION ( 'NONE',  ( -0.000000000000000000, 0.000000000000000000, -1.000000000000000000 ) ) ;
#16038=CARTESIAN_POINT ( 'NONE',  ( 0.000000000000000000, 0.000000000000000000, 60.90000000000001279 ) ) ;
#16066=ADVANCED_FACE ( 'NONE', ( #28048, #1212 ), #3393, .T. ) ;
#16113=EDGE_CURVE ( 'NONE', #31925, #2504, #2790, .T. ) ;
#16185=DIRECTION ( 'NONE',  ( -1.000000000000000000, 0.000000000000000000, 0.000000000000000000 ) ) ;
#16197=ORIENTED_EDGE ( 'NONE', *, *, #35060, .T. ) ;
#16216=ORIENTED_EDGE ( 'NONE', *, *, #29747, .F. ) ;
#16242=CARTESIAN_POINT ( 'NONE',  ( 4.000000000000000000, 4.898587196589412829E-16, 65.00000000000000000 ) ) ;
#16244=AXIS2_PLACEMENT_3D ( 'NONE', #26159, #12478, #23267 ) ;
#16252=CARTESIAN_POINT ( 'NONE',  ( 0.000000000000000000, 0.000000000000000000, -55.89999999999999858 ) ) ;
#16277=CARTESIAN_POINT ( 'NONE',  ( 5.400000000000071410, 0.9999999999999662492, -52.50000000000000000 ) ) ;
#16351=DIRECTION ( 'NONE',  ( 1.000000000000000000, 0.000000000000000000, 0.000000000000000000 ) ) ;
#16363=CARTESIAN_POINT ( 'NONE',  ( -4.000000000000000000, 0.000000000000000000, -32.00000000000000000 ) ) ;
#16388=CYLINDRICAL_SURFACE ( 'NONE', #11638, 4.000000000000000000 ) ;
#16391=AXIS2_PLACEMENT_3D ( 'NONE', #17332, #34098, #11955 ) ;
#16430=CARTESIAN_POINT ( 'NONE',  ( 3.799999999999999822, 0.000000000000000000, -40.89999999999999858 ) ) ;
#16445=AXIS2_PLACEMENT_3D ( 'NONE', #15328, #31377, #9233 ) ;
#16446=CIRCLE ( 'NONE', #11301, 4.000000000000000000 ) ;
#16448=ORIENTED_EDGE ( 'NONE', *, *, #30333, .F. ) ;
#16460=DIRECTION ( 'NONE',  ( -0.000000000000000000, 0.000000000000000000, -1.000000000000000000 ) ) ;
#16537=VECTOR ( 'NONE', #22568, 1000.000000000000000 ) ;
#16563=ORIENTED_EDGE ( 'NONE', *, *, #31321, .F. ) ;
#16605=AXIS2_PLACEMENT_3D ( 'NONE', #6303, #3268, #28451 ) ;
#16628=ORIENTED_EDGE ( 'NONE', *, *, #14341, .F. ) ;
#16632=CARTESIAN_POINT ( 'NONE',  ( 3.872983346207489852, 0.9999999999999522604, 65.00000000000000000 ) ) ;
#16641=CARTESIAN_POINT ( 'NONE',  ( -4.000000000000000000, 0.000000000000000000, 65.00000000000000000 ) ) ;
#16650=ADVANCED_FACE ( 'NONE', ( #31406 ), #23485, .T. ) ;
#16656=CARTESIAN_POINT ( 'NONE',  ( 3.872983346207489852, 0.9999999999999522604, -52.49999999999999289 ) ) ;
#16678=CARTESIAN_POINT ( 'NONE',  ( 9.714451465470119729E-14, 0.9999999999999870104, -44.50000000000000000 ) ) ;
#16709=CARTESIAN_POINT ( 'NONE',  ( 0.000000000000000000, 0.000000000000000000, -53.39999999999999858 ) ) ;
#16719=EDGE_CURVE ( 'NONE', #33549, #28168, #12688, .T. ) ;
#16724=ORIENTED_EDGE ( 'NONE', *, *, #17852, .F. ) ;
#16728=VERTEX_POINT ( 'NONE', #9975 ) ;
#16732=AXIS2_PLACEMENT_3D ( 'NONE', #23389, #9708, #17970 ) ;
#16751=ORIENTED_EDGE ( 'NONE', *, *, #23119, .F. ) ;
#16775=EDGE_CURVE ( 'NONE', #14055, #5329, #18903, .T. ) ;
#16806=ADVANCED_FACE ( 'NONE', ( #13395 ), #27445, .T. ) ;
#16809=CARTESIAN_POINT ( 'NONE',  ( 0.000000000000000000, 0.000000000000000000, -55.00000000000000000 ) ) ;
#16840=AXIS2_PLACEMENT_3D ( 'NONE', #19910, #19564, #20096 ) ;
#16850=ORIENTED_EDGE ( 'NONE', *, *, #34210, .T. ) ;
#16865=CARTESIAN_POINT ( 'NONE',  ( 3.799999999999999822, 0.000000000000000000, -55.89999999999999858 ) ) ;
#16872=EDGE_CURVE ( 'NONE', #26146, #33209, #5304, .T. ) ;
#16893=FACE_OUTER_BOUND ( 'NONE', #762, .T. ) ;
#16928=ORIENTED_EDGE ( 'NONE', *, *, #30333, .T. ) ;
#16935=CARTESIAN_POINT ( 'NONE',  ( 5.400000000000085620, -1.000000000000049516, 45.00000000000000711 ) ) ;
#16980=AXIS2_PLACEMENT_3D ( 'NONE', #26155, #4033, #34452 ) ;
#17018=PLANE ( 'NONE',  #4046 ) ;
#17029=VERTEX_POINT ( 'NONE', #14086 ) ;
#17045=LINE ( 'NONE', #16865, #27232 ) ;
#17105=ORIENTED_EDGE ( 'NONE', *, *, #17350, .F. ) ;
#17133=VECTOR ( 'NONE', #18528, 1000.000000000000000 ) ;
#17153=DIRECTION ( 'NONE',  ( 1.000000000000000000, 0.000000000000000000, 0.000000000000000000 ) ) ;
#17189=EDGE_CURVE ( 'NONE', #19003, #1732, #26416, .T. ) ;
#17197=EDGE_CURVE ( 'NONE', #31889, #14055, #34446, .T. ) ;
#17202=EDGE_LOOP ( 'NONE', ( #30130, #23241, #11922, #16928, #31038 ) ) ;
#17211=CIRCLE ( 'NONE', #33320, 3.799999999999999822 ) ;
#17212=CARTESIAN_POINT ( 'NONE',  ( 0.000000000000000000, 0.000000000000000000, -55.89999999999999858 ) ) ;
#17213=DIRECTION ( 'NONE',  ( 0.000000000000000000, 0.000000000000000000, 1.000000000000000000 ) ) ;
#17237=CARTESIAN_POINT ( 'NONE',  ( 4.000000000000000000, 4.898587196589412829E-16, -55.00000000000000000 ) ) ;
#17238=EDGE_CURVE ( 'NONE', #17029, #21809, #34616, .T. ) ;
#17255=DIRECTION ( 'NONE',  ( 0.000000000000000000, 0.000000000000000000, -1.000000000000000000 ) ) ;
#17272=CARTESIAN_POINT ( 'NONE',  ( 0.000000000000000000, 0.000000000000000000, -55.89999999999999858 ) ) ;
#17277=CARTESIAN_POINT ( 'NONE',  ( 0.000000000000000000, 0.000000000000000000, -55.89999999999999858 ) ) ;
#17280=CARTESIAN_POINT ( 'NONE',  ( 0.000000000000000000, 0.000000000000000000, -52.50000000000000000 ) ) ;
#17290=VERTEX_POINT ( 'NONE', #32264 ) ;
#17332=CARTESIAN_POINT ( 'NONE',  ( 0.000000000000000000, 0.000000000000000000, -65.00000000000000000 ) ) ;
#17350=EDGE_CURVE ( 'NONE', #529, #19681, #17211, .T. ) ;
#17358=ADVANCED_FACE ( 'NONE', ( #9884 ), #20848, .F. ) ;
#17363=EDGE_CURVE ( 'NONE', #9289, #15509, #29889, .T. ) ;
#17384=VERTEX_POINT ( 'NONE', #27352 ) ;
#17449=CARTESIAN_POINT ( 'NONE',  ( 0.000000000000000000, 0.000000000000000000, 60.00000000000000000 ) ) ;
#17504=CARTESIAN_POINT ( 'NONE',  ( 4.000000000000000000, 4.898587196589412829E-16, -40.89999999999999858 ) ) ;
#17513=DIRECTION ( 'NONE',  ( 0.000000000000000000, 0.000000000000000000, -1.000000000000000000 ) ) ;
#17514=CARTESIAN_POINT ( 'NONE',  ( 0.000000000000000000, 0.000000000000000000, 65.00000000000000000 ) ) ;
#17540=ORIENTED_EDGE ( 'NONE', *, *, #21841, .T. ) ;
#17548=CARTESIAN_POINT ( 'NONE',  ( 5.400000000000085620, -1.000000000000049516, -44.50000000000000000 ) ) ;
#17579=ADVANCED_FACE ( 'NONE', ( #11483 ), #24997, .T. ) ;
#17589=CARTESIAN_POINT ( 'NONE',  ( 9.714451465470119729E-14, 0.9999999999999870104, -40.00000000000000000 ) ) ;
#17607=VECTOR ( 'NONE', #24190, 1000.000000000000000 ) ;
#17651=VERTEX_POINT ( 'NONE', #22454 ) ;
#17701=DIRECTION ( 'NONE',  ( -1.000000000000000000, 0.000000000000000000, 0.000000000000000000 ) ) ;
#17706=VERTEX_POINT ( 'NONE', #22988 ) ;
#17804=VECTOR ( 'NONE', #9145, 1000.000000000000000 ) ;
#17807=DIRECTION ( 'NONE',  ( 1.000000000000000000, 0.000000000000000000, 0.000000000000000000 ) ) ;
#17816=LINE ( 'NONE', #9368, #20936 ) ;
#17838=VERTEX_POINT ( 'NONE', #31105 ) ;
#17851=CARTESIAN_POINT ( 'NONE',  ( 0.000000000000000000, 0.000000000000000000, 60.00000000000000000 ) ) ;
#17852=EDGE_CURVE ( 'NONE', #35528, #8976, #22259, .T. ) ;
#17875=CARTESIAN_POINT ( 'NONE',  ( 0.000000000000000000, 0.000000000000000000, 35.10000000000000142 ) ) ;
#17890=VECTOR ( 'NONE', #7177, 1000.000000000000000 ) ;
#17930=CARTESIAN_POINT ( 'NONE',  ( 3.872983346207517386, -1.000000000000028644, -52.50000000000000000 ) ) ;
#17970=DIRECTION ( 'NONE',  ( -1.000000000000000000, 0.000000000000000000, 0.000000000000000000 ) ) ;
#17977=VECTOR ( 'NONE', #31204, 1000.000000000000000 ) ;
#17982=VECTOR ( 'NONE', #14818, 1000.000000000000000 ) ;
#17995=DIRECTION ( 'NONE',  ( 0.000000000000000000, 0.000000000000000000, -1.000000000000000000 ) ) ;
#18042=DIRECTION ( 'NONE',  ( -1.000000000000000000, 0.000000000000000000, 0.000000000000000000 ) ) ;
#18063=SHAPE_REPRESENTATION ( 'shaft 3', ( #21307 ), #26556 ) ;
#18082=PLANE ( 'NONE',  #23378 ) ;
#18103=ORIENTED_EDGE ( 'NONE', *, *, #5498, .T. ) ;
#18119=CIRCLE ( 'NONE', #16391, 4.000000000000000000 ) ;
#18122=AXIS2_PLACEMENT_3D ( 'NONE', #17212, #1889, #9306 ) ;
#18134=ORIENTED_EDGE ( 'NONE', *, *, #33890, .T. ) ;
#18138=EDGE_CURVE ( 'NONE', #17029, #19012, #33237, .T. ) ;
#18143=DIRECTION ( 'NONE',  ( -1.000000000000000000, 0.000000000000000000, 0.000000000000000000 ) ) ;
#18156=VERTEX_POINT ( 'NONE', #16656 ) ;
#18192=EDGE_LOOP ( 'NONE', ( #12710, #26529 ) ) ;
#18207=CIRCLE ( 'NONE', #34305, 3.799999999999999822 ) ;
#18213=DIRECTION ( 'NONE',  ( 1.000000000000000000, -1.110223024625156540E-16, 0.000000000000000000 ) ) ;
#18245=AXIS2_PLACEMENT_3D ( 'NONE', #21525, #32524, #24616 ) ;
#18254=CARTESIAN_POINT ( 'NONE',  ( 0.000000000000000000, 0.000000000000000000, 65.00000000000000000 ) ) ;
#18260=ORIENTED_EDGE ( 'NONE', *, *, #8321, .T. ) ;
#18267=ORIENTED_EDGE ( 'NONE', *, *, #34873, .F. ) ;
#18279=AXIS2_PLACEMENT_3D ( 'NONE', #11864, #4317, #15083 ) ;
#18283=AXIS2_PLACEMENT_3D ( 'NONE', #8937, #17213, #28221 ) ;
#18284=SURFACE_SIDE_STYLE ('',( #9825 ) ) ;
#18292=DIRECTION ( 'NONE',  ( 1.000000000000000000, 0.000000000000000000, 0.000000000000000000 ) ) ;
#18295=CARTESIAN_POINT ( 'NONE',  ( 4.000000000000000000, 4.898587196589412829E-16, 60.00000000000000000 ) ) ;
#18318=DIRECTION ( 'NONE',  ( -1.000000000000000000, 0.000000000000000000, 0.000000000000000000 ) ) ;
#18333=ORIENTED_EDGE ( 'NONE', *, *, #7492, .F. ) ;
#18334=AXIS2_PLACEMENT_3D ( 'NONE', #19456, #548, #33491 ) ;
#18340=DIRECTION ( 'NONE',  ( -0.000000000000000000, 0.000000000000000000, -1.000000000000000000 ) ) ;
#18346=ORIENTED_EDGE ( 'NONE', *, *, #12808, .F. ) ;
#18353=VECTOR ( 'NONE', #24424, 1000.000000000000000 ) ;
#18355=DIRECTION ( 'NONE',  ( -1.000000000000000000, 0.000000000000000000, 0.000000000000000000 ) ) ;
#18361=VECTOR ( 'NONE', #18213, 1000.000000000000000 ) ;
#18372=ORIENTED_EDGE ( 'NONE', *, *, #28415, .T. ) ;
#18403=AXIS2_PLACEMENT_3D ( 'NONE', #18254, #20593, #14843 ) ;
#18409=PLANE ( 'NONE',  #10701 ) ;
#18417=DIRECTION ( 'NONE',  ( -1.000000000000000000, 0.000000000000000000, 0.000000000000000000 ) ) ;
#18470=ORIENTED_EDGE ( 'NONE', *, *, #32128, .F. ) ;
#18473=CARTESIAN_POINT ( 'NONE',  ( 4.000000000000000000, 4.898587196589412829E-16, 65.00000000000000000 ) ) ;
#18475=VERTEX_POINT ( 'NONE', #21442 ) ;
#18524=ORIENTED_EDGE ( 'NONE', *, *, #22916, .F. ) ;
#18525=DIRECTION ( 'NONE',  ( -1.000000000000000000, 0.000000000000000000, 0.000000000000000000 ) ) ;
#18528=DIRECTION ( 'NONE',  ( 0.000000000000000000, 0.000000000000000000, -1.000000000000000000 ) ) ;
#18547=VERTEX_POINT ( 'NONE', #28102 ) ;
#18552=ADVANCED_FACE ( 'NONE', ( #30619 ), #8479, .T. ) ;
#18553=VECTOR ( 'NONE', #8129, 1000.000000000000000 ) ;
#18554=AXIS2_PLACEMENT_3D ( 'NONE', #20056, #22948, #20229 ) ;
#18555=ADVANCED_FACE ( 'NONE', ( #33322, #8817 ), #19779, .F. ) ;
#18586=CARTESIAN_POINT ( 'NONE',  ( -4.000000000000000000, 0.000000000000000000, 65.00000000000000000 ) ) ;
#18598=CARTESIAN_POINT ( 'NONE',  ( -3.799999999999999822, 4.653657836759942730E-16, -55.89999999999999858 ) ) ;
#18625=CARTESIAN_POINT ( 'NONE',  ( 0.000000000000000000, 0.000000000000000000, -55.89999999999999858 ) ) ;
#18630=CARTESIAN_POINT ( 'NONE',  ( 4.000000000000000000, 4.898587196589412829E-16, 45.00000000000000711 ) ) ;
#18642=EDGE_LOOP ( 'NONE', ( #4652, #18470 ) ) ;
#18649=ADVANCED_FACE ( 'NONE', ( #6132, #719 ), #19963, .T. ) ;
#18672=ORIENTED_EDGE ( 'NONE', *, *, #25604, .F. ) ;
#18708=EDGE_LOOP ( 'NONE', ( #32336, #29635 ) ) ;
#18775=ORIENTED_EDGE ( 'NONE', *, *, #10968, .F. ) ;
#18776=AXIS2_PLACEMENT_3D ( 'NONE', #13455, #24437, #35422 ) ;
#18835=EDGE_LOOP ( 'NONE', ( #32120, #7605 ) ) ;
#18842=EDGE_CURVE ( 'NONE', #891, #5174, #5653, .T. ) ;
#18856=VECTOR ( 'NONE', #22308, 1000.000000000000000 ) ;
#18864=CARTESIAN_POINT ( 'NONE',  ( 5.400000000000085620, -1.000000000000049516, -32.00000000000000000 ) ) ;
#18865=ORIENTED_EDGE ( 'NONE', *, *, #17238, .T. ) ;
#18879=MECHANICAL_DESIGN_GEOMETRIC_PRESENTATION_REPRESENTATION('',(#29742),#7879);
#18887=CYLINDRICAL_SURFACE ( 'NONE', #163, 4.000000000000000000 ) ;
#18893=DIRECTION ( 'NONE',  ( 0.000000000000000000, 0.000000000000000000, 1.000000000000000000 ) ) ;
#18903=CIRCLE ( 'NONE', #28110, 4.000000000000000000 ) ;
#18949=CARTESIAN_POINT ( 'NONE',  ( 0.000000000000000000, 0.000000000000000000, -53.39999999999999858 ) ) ;
#18955=PRODUCT_DEFINITION_FORMATION_WITH_SPECIFIED_SOURCE ( 'ANY', '', #6342, .NOT_KNOWN. ) ;
#18970=EDGE_CURVE ( 'NONE', #15000, #30905, #10794, .T. ) ;
#18978=ORIENTED_EDGE ( 'NONE', *, *, #4845, .F. ) ;
#19003=VERTEX_POINT ( 'NONE', #18295 ) ;
#19012=VERTEX_POINT ( 'NONE', #17930 ) ;
#19043=DIRECTION ( 'NONE',  ( 1.000000000000000000, -1.110223024625156540E-16, 0.000000000000000000 ) ) ;
#19063=DIRECTION ( 'NONE',  ( 0.000000000000000000, 0.000000000000000000, -1.000000000000000000 ) ) ;
#19077=MECHANICAL_DESIGN_GEOMETRIC_PRESENTATION_REPRESENTATION('',(#30571),#31725);
#19110=FACE_OUTER_BOUND ( 'NONE', #21680, .T. ) ;
#19129=ORIENTED_EDGE ( 'NONE', *, *, #23644, .T. ) ;
#19160=CARTESIAN_POINT ( 'NONE',  ( 3.872983346207517386, -1.000000000000028644, -32.00000000000000000 ) ) ;
#19211=ADVANCED_FACE ( 'NONE', ( #2299 ), #8369, .T. ) ;
#19216=ORIENTED_EDGE ( 'NONE', *, *, #9739, .T. ) ;
#19255=ORIENTED_EDGE ( 'NONE', *, *, #31053, .F. ) ;
#19261=ORIENTED_EDGE ( 'NONE', *, *, #23155, .F. ) ;
#19285=ORIENTED_EDGE ( 'NONE', *, *, #34210, .F. ) ;
#19295=VERTEX_POINT ( 'NONE', #5512 ) ;
#19299=ORIENTED_EDGE ( 'NONE', *, *, #5962, .F. ) ;
#19325=AXIS2_PLACEMENT_3D ( 'NONE', #17277, #201, #25232 ) ;
#19326=AXIS2_PLACEMENT_3D ( 'NONE', #26080, #9688, #1411 ) ;
#19345=AXIS2_PLACEMENT_3D ( 'NONE', #5744, #30580, #5913 ) ;
#19347=ORIENTED_EDGE ( 'NONE', *, *, #11069, .F. ) ;
#19354=AXIS2_PLACEMENT_3D ( 'NONE', #12450, #31179, #28481 ) ;
#19394=AXIS2_PLACEMENT_3D ( 'NONE', #27992, #3687, #30866 ) ;
#19408=DIRECTION ( 'NONE',  ( 0.000000000000000000, 0.000000000000000000, 1.000000000000000000 ) ) ;
#19422=DIRECTION ( 'NONE',  ( 0.000000000000000000, 0.000000000000000000, -1.000000000000000000 ) ) ;
#19433=AXIS2_PLACEMENT_3D ( 'NONE', #1680, #7066, #18042 ) ;
#19456=CARTESIAN_POINT ( 'NONE',  ( 0.000000000000000000, 0.000000000000000000, -43.60000000000000142 ) ) ;
#19504=ORIENTED_EDGE ( 'NONE', *, *, #2300, .F. ) ;
#19539=CARTESIAN_POINT ( 'NONE',  ( 0.000000000000000000, 0.000000000000000000, -55.00000000000000000 ) ) ;
#19546=ADVANCED_FACE ( 'NONE', ( #6963 ), #21179, .T. ) ;
#19554=VECTOR ( 'NONE', #8350, 1000.000000000000000 ) ;
#19564=DIRECTION ( 'NONE',  ( -0.000000000000000000, 0.000000000000000000, -1.000000000000000000 ) ) ;
#19582=CARTESIAN_POINT ( 'NONE',  ( 3.872983346207489852, 0.9999999999999522604, -40.00000000000000000 ) ) ;
#19595=AXIS2_PLACEMENT_3D ( 'NONE', #7333, #4475, #12915 ) ;
#19597=CARTESIAN_POINT ( 'NONE',  ( -3.799999999999999822, 4.653657836759942730E-16, -32.00000000000000000 ) ) ;
#19605=AXIS2_PLACEMENT_3D ( 'NONE', #31532, #26496, #26130 ) ;
#19628=EDGE_CURVE ( 'NONE', #10539, #18156, #35240, .T. ) ;
#19675=DIRECTION ( 'NONE',  ( -1.000000000000000000, 0.000000000000000000, 0.000000000000000000 ) ) ;
#19678=CARTESIAN_POINT ( 'NONE',  ( 5.400000000000071410, 0.9999999999999662492, -40.00000000000000000 ) ) ;
#19681=VERTEX_POINT ( 'NONE', #15759 ) ;
#19716=UNCERTAINTY_MEASURE_WITH_UNIT (LENGTH_MEASURE( 1.000000000000000082E-05 ), #26510, 'distance_accuracy_value', 'NONE');
#19717=APPLICATION_CONTEXT ( 'automotive_design' ) ;
#19768=ORIENTED_EDGE ( 'NONE', *, *, #18842, .T. ) ;
#19779=PLANE ( 'NONE',  #33785 ) ;
#19824=VECTOR ( 'NONE', #20248, 1000.000000000000000 ) ;
#19864=DIRECTION ( 'NONE',  ( -1.000000000000000000, 0.000000000000000000, 0.000000000000000000 ) ) ;
#19873=CARTESIAN_POINT ( 'NONE',  ( 0.000000000000000000, 0.000000000000000000, 65.00000000000000000 ) ) ;
#19906=DIRECTION ( 'NONE',  ( 0.000000000000000000, 0.000000000000000000, -1.000000000000000000 ) ) ;
#19910=CARTESIAN_POINT ( 'NONE',  ( 0.000000000000000000, 0.000000000000000000, 65.00000000000000000 ) ) ;
#19912=DIRECTION ( 'NONE',  ( 1.000000000000000000, 0.000000000000000000, 0.000000000000000000 ) ) ;
#19943=AXIS2_PLACEMENT_3D ( 'NONE', #31817, #12922, #21189 ) ;
#19963=PLANE ( 'NONE',  #18334 ) ;
#19971=DIRECTION ( 'NONE',  ( 1.000000000000000000, 0.000000000000000000, 0.000000000000000000 ) ) ;
#20046=ADVANCED_FACE ( 'NONE', ( #31410 ), #31765, .T. ) ;
#20056=CARTESIAN_POINT ( 'NONE',  ( 0.000000000000000000, 0.000000000000000000, -53.39999999999999858 ) ) ;
#20057=VECTOR ( 'NONE', #28848, 1000.000000000000000 ) ;
#20096=DIRECTION ( 'NONE',  ( -1.000000000000000000, 0.000000000000000000, 0.000000000000000000 ) ) ;
#20119=ORIENTED_EDGE ( 'NONE', *, *, #21511, .T. ) ;
#20125=VERTEX_POINT ( 'NONE', #4777 ) ;
#20129=EDGE_LOOP ( 'NONE', ( #6338, #24724 ) ) ;
#20198=LINE ( 'NONE', #31029, #26777 ) ;
#20202=ADVANCED_FACE ( 'NONE', ( #35371 ), #27091, .T. ) ;
#20229=DIRECTION ( 'NONE',  ( 1.000000000000000000, 0.000000000000000000, 0.000000000000000000 ) ) ;
#20248=DIRECTION ( 'NONE',  ( 0.000000000000000000, 1.000000000000000000, 0.000000000000000000 ) ) ;
#20254=DIRECTION ( 'NONE',  ( -1.000000000000000000, 0.000000000000000000, 0.000000000000000000 ) ) ;
#20354=ORIENTED_EDGE ( 'NONE', *, *, #17363, .F. ) ;
#20422=CARTESIAN_POINT ( 'NONE',  ( 0.000000000000000000, 0.000000000000000000, -40.89999999999999858 ) ) ;
#20426=CARTESIAN_POINT ( 'NONE',  ( 0.000000000000000000, 0.000000000000000000, -44.50000000000000000 ) ) ;
#20434=VECTOR ( 'NONE', #26352, 1000.000000000000000 ) ;
#20464=CARTESIAN_POINT ( 'NONE',  ( 5.400000000000071410, 0.9999999999999662492, -32.00000000000000000 ) ) ;
#20506=VECTOR ( 'NONE', #8225, 1000.000000000000000 ) ;
#20511=DIRECTION ( 'NONE',  ( 1.000000000000000000, 0.000000000000000000, 0.000000000000000000 ) ) ;
#20567=CARTESIAN_POINT ( 'NONE',  ( 5.400000000000071410, 0.9999999999999662492, -44.50000000000000000 ) ) ;
#20590=CARTESIAN_POINT ( 'NONE',  ( 0.000000000000000000, 0.000000000000000000, 65.00000000000000000 ) ) ;
#20593=DIRECTION ( 'NONE',  ( -0.000000000000000000, 0.000000000000000000, -1.000000000000000000 ) ) ;
#20615=FACE_OUTER_BOUND ( 'NONE', #8096, .T. ) ;
#20651=AXIS2_PLACEMENT_3D ( 'NONE', #1804, #31852, #29171 ) ;
#20699=FACE_OUTER_BOUND ( 'NONE', #24555, .T. ) ;
#20745=EDGE_CURVE ( 'NONE', #31797, #3997, #2394, .T. ) ;
#20748=ORIENTED_EDGE ( 'NONE', *, *, #9739, .F. ) ;
#20755=EDGE_LOOP ( 'NONE', ( #32339, #5037 ) ) ;
#20761=CARTESIAN_POINT ( 'NONE',  ( -4.000000000000000000, 0.000000000000000000, 65.00000000000000000 ) ) ;
#20848=PLANE ( 'NONE',  #20651 ) ;
#20849=VECTOR ( 'NONE', #7773, 1000.000000000000000 ) ;
#20873=EDGE_LOOP ( 'NONE', ( #14433, #25967, #16628, #33845 ) ) ;
#20936=VECTOR ( 'NONE', #28645, 1000.000000000000000 ) ;
#20958=DIRECTION ( 'NONE',  ( -1.000000000000000000, 0.000000000000000000, 0.000000000000000000 ) ) ;
#20961=FACE_OUTER_BOUND ( 'NONE', #13859, .T. ) ;
#20987=CARTESIAN_POINT ( 'NONE',  ( 9.714451465470119729E-14, 0.9999999999999870104, 53.00000000000000711 ) ) ;
#21003=PLANE ( 'NONE',  #4910 ) ;
#21049=CYLINDRICAL_SURFACE ( 'NONE', #12898, 3.799999999999999822 ) ;
#21056=VECTOR ( 'NONE', #8568, 1000.000000000000000 ) ;
#21076=ADVANCED_FACE ( 'NONE', ( #31064 ), #14480, .T. ) ;
#21079=ORIENTED_EDGE ( 'NONE', *, *, #9978, .F. ) ;
#21080=CARTESIAN_POINT ( 'NONE',  ( -4.000000000000000000, 0.000000000000000000, 65.00000000000000000 ) ) ;
#21148=CARTESIAN_POINT ( 'NONE',  ( 0.000000000000000000, 0.000000000000000000, -31.10000000000000142 ) ) ;
#21168=ADVANCED_FACE ( 'NONE', ( #22767 ), #9098, .T. ) ;
#21175=CARTESIAN_POINT ( 'NONE',  ( -4.000000000000000000, 0.000000000000000000, -53.39999999999999858 ) ) ;
#21179=PLANE ( 'NONE',  #32133 ) ;
#21189=DIRECTION ( 'NONE',  ( 1.000000000000000000, 0.000000000000000000, 0.000000000000000000 ) ) ;
#21191=CARTESIAN_POINT ( 'NONE',  ( 0.000000000000000000, 0.000000000000000000, -32.00000000000000000 ) ) ;
#21208=ORIENTED_EDGE ( 'NONE', *, *, #63, .T. ) ;
#21231=DIRECTION ( 'NONE',  ( 0.000000000000000000, 0.000000000000000000, -1.000000000000000000 ) ) ;
#21252=CYLINDRICAL_SURFACE ( 'NONE', #13668, 4.000000000000000000 ) ;
#21253=ORIENTED_EDGE ( 'NONE', *, *, #34838, .F. ) ;
#21282=LINE ( 'NONE', #34459, #20434 ) ;
#21297=ORIENTED_EDGE ( 'NONE', *, *, #4897, .T. ) ;
#21307=AXIS2_PLACEMENT_3D ( 'NONE', #26589, #12725, #18292 ) ;
#21317=CARTESIAN_POINT ( 'NONE',  ( -3.799999999999999822, 4.653657836759942730E-16, 60.00000000000000000 ) ) ;
#21365=LINE ( 'NONE', #7156, #11308 ) ;
#21406=CARTESIAN_POINT ( 'NONE',  ( -4.000000000000000000, 0.000000000000000000, 65.00000000000000000 ) ) ;
#21421=CARTESIAN_POINT ( 'NONE',  ( 5.400000000000085620, -1.000000000000049516, -44.50000000000000000 ) ) ;
#21442=CARTESIAN_POINT ( 'NONE',  ( 3.799999999999999822, 0.000000000000000000, -55.00000000000000000 ) ) ;
#21452=CARTESIAN_POINT ( 'NONE',  ( 4.000000000000000000, 4.898587196589412829E-16, 65.00000000000000000 ) ) ;
#21464=CARTESIAN_POINT ( 'NONE',  ( 0.000000000000000000, 0.000000000000000000, -40.00000000000000711 ) ) ;
#21469=LINE ( 'NONE', #15713, #23292 ) ;
#21479=CARTESIAN_POINT ( 'NONE',  ( 0.000000000000000000, 0.000000000000000000, 65.00000000000000000 ) ) ;
#21483=DIRECTION ( 'NONE',  ( 0.000000000000000000, 0.000000000000000000, -1.000000000000000000 ) ) ;
#21511=EDGE_CURVE ( 'NONE', #14882, #20125, #15144, .T. ) ;
#21525=CARTESIAN_POINT ( 'NONE',  ( 0.000000000000000000, 0.000000000000000000, -40.89999999999999858 ) ) ;
#21527=FACE_OUTER_BOUND ( 'NONE', #12772, .T. ) ;
#21529=DIRECTION ( 'NONE',  ( 0.000000000000000000, 0.000000000000000000, 1.000000000000000000 ) ) ;
#21576=VERTEX_POINT ( 'NONE', #3492 ) ;
#21596=CARTESIAN_POINT ( 'NONE',  ( -4.000000000000000000, 0.000000000000000000, 65.00000000000000000 ) ) ;
#21625=LINE ( 'NONE', #18586, #20849 ) ;
#21627=AXIS2_PLACEMENT_3D ( 'NONE', #12249, #9545, #20511 ) ;
#21645=ORIENTED_EDGE ( 'NONE', *, *, #8591, .T. ) ;
#21680=EDGE_LOOP ( 'NONE', ( #16448, #8052, #18103, #6947 ) ) ;
#21683=ADVANCED_FACE ( 'NONE', ( #30326, #244 ), #33721, .F. ) ;
#21693=FACE_OUTER_BOUND ( 'NONE', #5944, .T. ) ;
#21694=CARTESIAN_POINT ( 'NONE',  ( 4.000000000000000000, 4.898587196589412829E-16, 60.90000000000001279 ) ) ;
#21711=CIRCLE ( 'NONE', #19433, 3.799999999999999822 ) ;
#21759=DIRECTION ( 'NONE',  ( -1.000000000000000000, 0.000000000000000000, 0.000000000000000000 ) ) ;
#21760=EDGE_LOOP ( 'NONE', ( #14869, #25420 ) ) ;
#21795=EDGE_CURVE ( 'NONE', #30905, #34581, #29034, .T. ) ;
#21802=CIRCLE ( 'NONE', #2311, 4.000000000000000000 ) ;
#21806=DIRECTION ( 'NONE',  ( -1.000000000000000000, 0.000000000000000000, 0.000000000000000000 ) ) ;
#21809=VERTEX_POINT ( 'NONE', #1308 ) ;
#21813=PLANE ( 'NONE',  #7094 ) ;
#21841=EDGE_CURVE ( 'NONE', #17706, #334, #32517, .T. ) ;
#21854=ORIENTED_EDGE ( 'NONE', *, *, #28476, .F. ) ;
#21865=LINE ( 'NONE', #16632, #6741 ) ;
#21866=CARTESIAN_POINT ( 'NONE',  ( 3.799999999999999822, 0.000000000000000000, 35.10000000000000142 ) ) ;
#21886=ADVANCED_FACE ( 'NONE', ( #12833 ), #23815, .T. ) ;
#21931=CARTESIAN_POINT ( 'NONE',  ( 0.000000000000000000, 0.000000000000000000, 35.10000000000000142 ) ) ;
#21946=ORIENTED_EDGE ( 'NONE', *, *, #21795, .T. ) ;
#21969=EDGE_CURVE ( 'NONE', #2504, #32249, #33146, .T. ) ;
#21993=AXIS2_PLACEMENT_3D ( 'NONE', #19873, #28362, #8560 ) ;
#21995=CARTESIAN_POINT ( 'NONE',  ( 3.872983346207517386, -1.000000000000028644, 55.00000000000000711 ) ) ;
#22032=FACE_OUTER_BOUND ( 'NONE', #170, .T. ) ;
#22035=DIRECTION ( 'NONE',  ( -1.000000000000000000, 0.000000000000000000, 0.000000000000000000 ) ) ;
#22039=ORIENTED_EDGE ( 'NONE', *, *, #10968, .T. ) ;
#22049=ORIENTED_EDGE ( 'NONE', *, *, #27833, .F. ) ;
#22085=DIRECTION ( 'NONE',  ( -1.000000000000000000, 1.110223024625156540E-16, 0.000000000000000000 ) ) ;
#22089=EDGE_CURVE ( 'NONE', #17290, #3282, #10708, .T. ) ;
#22115=DIRECTION ( 'NONE',  ( -1.000000000000000000, 0.000000000000000000, 0.000000000000000000 ) ) ;
#22173=ORIENTED_EDGE ( 'NONE', *, *, #26434, .F. ) ;
#22174=AXIS2_PLACEMENT_3D ( 'NONE', #21148, #31780, #20958 ) ;
#22259=CIRCLE ( 'NONE', #6740, 3.799999999999999822 ) ;
#22269=VECTOR ( 'NONE', #27113, 1000.000000000000000 ) ;
#22293=CIRCLE ( 'NONE', #457, 4.000000000000000000 ) ;
#22297=CARTESIAN_POINT ( 'NONE',  ( -3.799999999999999822, 4.653657836759942730E-16, 35.10000000000000142 ) ) ;
#22308=DIRECTION ( 'NONE',  ( -0.000000000000000000, 0.000000000000000000, -1.000000000000000000 ) ) ;
#22341=DIRECTION ( 'NONE',  ( 0.000000000000000000, 0.000000000000000000, -1.000000000000000000 ) ) ;
#22404=AXIS2_PLACEMENT_3D ( 'NONE', #8081, #19422, #22115 ) ;
#22419=CARTESIAN_POINT ( 'NONE',  ( 3.872983346207489852, 0.9999999999999522604, 45.00000000000000711 ) ) ;
#22431=AXIS2_PLACEMENT_3D ( 'NONE', #21191, #34361, #24097 ) ;
#22435=ORIENTED_EDGE ( 'NONE', *, *, #14296, .F. ) ;
#22436=ORIENTED_EDGE ( 'NONE', *, *, #18138, .T. ) ;
#22454=CARTESIAN_POINT ( 'NONE',  ( 5.400000000000085620, -1.000000000000049516, 55.00000000000000711 ) ) ;
#22461=EDGE_CURVE ( 'NONE', #8976, #35528, #22526, .T. ) ;
#22488=ORIENTED_EDGE ( 'NONE', *, *, #14000, .T. ) ;
#22525=EDGE_LOOP ( 'NONE', ( #7414, #10916, #8198, #19285 ) ) ;
#22526=CIRCLE ( 'NONE', #33456, 3.799999999999999822 ) ;
#22562=AXIS2_PLACEMENT_3D ( 'NONE', #30134, #8328, #28098 ) ;
#22568=DIRECTION ( 'NONE',  ( -0.000000000000000000, 0.000000000000000000, -1.000000000000000000 ) ) ;
#22572=VERTEX_POINT ( 'NONE', #29081 ) ;
#22602=ORIENTED_EDGE ( 'NONE', *, *, #8364, .T. ) ;
#22604=VECTOR ( 'NONE', #31565, 1000.000000000000000 ) ;
#22626=VECTOR ( 'NONE', #16012, 1000.000000000000000 ) ;
#22678=AXIS2_PLACEMENT_3D ( 'NONE', #20426, #23512, #20254 ) ;
#22708=EDGE_LOOP ( 'NONE', ( #9548, #5242, #26099, #18775 ) ) ;
#22720=VECTOR ( 'NONE', #25519, 1000.000000000000000 ) ;
#22737=FACE_OUTER_BOUND ( 'NONE', #10808, .T. ) ;
#22767=FACE_OUTER_BOUND ( 'NONE', #12793, .T. ) ;
#22791=CARTESIAN_POINT ( 'NONE',  ( 0.000000000000000000, 0.000000000000000000, 65.00000000000000000 ) ) ;
#22847=DIRECTION ( 'NONE',  ( 0.000000000000000000, 0.000000000000000000, 1.000000000000000000 ) ) ;
#22867=LINE ( 'NONE', #33864, #3716 ) ;
#22892=CARTESIAN_POINT ( 'NONE',  ( 0.000000000000000000, 0.000000000000000000, -53.39999999999999858 ) ) ;
#22916=EDGE_CURVE ( 'NONE', #7584, #18156, #1869, .T. ) ;
#22917=ORIENTED_EDGE ( 'NONE', *, *, #18842, .F. ) ;
#22925=VECTOR ( 'NONE', #2603, 1000.000000000000000 ) ;
#22940=DIRECTION ( 'NONE',  ( 0.000000000000000000, 0.000000000000000000, -1.000000000000000000 ) ) ;
#22948=DIRECTION ( 'NONE',  ( 0.000000000000000000, 0.000000000000000000, 1.000000000000000000 ) ) ;
#22968=( LENGTH_UNIT ( ) NAMED_UNIT ( * ) SI_UNIT ( .MILLI., .METRE. ) );
#22988=CARTESIAN_POINT ( 'NONE',  ( -3.799999999999999822, 4.653657836759942730E-16, -52.50000000000000000 ) ) ;
#22996=DIRECTION ( 'NONE',  ( 0.000000000000000000, 0.000000000000000000, 1.000000000000000000 ) ) ;
#22998=CARTESIAN_POINT ( 'NONE',  ( 0.000000000000000000, 0.000000000000000000, -32.00000000000000000 ) ) ;
#23017=ORIENTED_EDGE ( 'NONE', *, *, #30126, .F. ) ;
#23044=FACE_BOUND ( 'NONE', #10558, .T. ) ;
#23105=EDGE_LOOP ( 'NONE', ( #33125, #19261 ) ) ;
#23119=EDGE_CURVE ( 'NONE', #9483, #3997, #32629, .T. ) ;
#23150=( NAMED_UNIT ( * ) SI_UNIT ( $, .STERADIAN. ) SOLID_ANGLE_UNIT ( ) );
#23155=EDGE_CURVE ( 'NONE', #2210, #33416, #27768, .T. ) ;
#23159=AXIS2_PLACEMENT_3D ( 'NONE', #18625, #35210, #2620 ) ;
#23241=ORIENTED_EDGE ( 'NONE', *, *, #8821, .F. ) ;
#23250=VERTEX_POINT ( 'NONE', #29344 ) ;
#23267=DIRECTION ( 'NONE',  ( -1.000000000000000000, 0.000000000000000000, 0.000000000000000000 ) ) ;
#23268=CARTESIAN_POINT ( 'NONE',  ( 4.000000000000000000, 4.898587196589412829E-16, 65.00000000000000000 ) ) ;
#23292=VECTOR ( 'NONE', #32465, 1000.000000000000000 ) ;
#23335=AXIS2_PLACEMENT_3D ( 'NONE', #30856, #14990, #17153 ) ;
#23345=DIRECTION ( 'NONE',  ( -1.000000000000000000, 1.110223024625156540E-16, 0.000000000000000000 ) ) ;
#23363=CARTESIAN_POINT ( 'NONE',  ( 1.110223024625156540E-13, -1.000000000000042633, -40.00000000000000000 ) ) ;
#23375=CARTESIAN_POINT ( 'NONE',  ( 0.000000000000000000, 0.000000000000000000, 35.10000000000000142 ) ) ;
#23378=AXIS2_PLACEMENT_3D ( 'NONE', #4255, #23500, #29445 ) ;
#23389=CARTESIAN_POINT ( 'NONE',  ( 0.000000000000000000, 0.000000000000000000, 60.00000000000000000 ) ) ;
#23400=AXIS2_PLACEMENT_3D ( 'NONE', #15877, #5286, #26902 ) ;
#23414=DIRECTION ( 'NONE',  ( 0.000000000000000000, 0.000000000000000000, -1.000000000000000000 ) ) ;
#23436=VECTOR ( 'NONE', #6945, 1000.000000000000000 ) ;
#23450=DIRECTION ( 'NONE',  ( -1.000000000000000000, 0.000000000000000000, 0.000000000000000000 ) ) ;
#23457=DIRECTION ( 'NONE',  ( 0.000000000000000000, 1.000000000000000000, 0.000000000000000000 ) ) ;
#23471=DIRECTION ( 'NONE',  ( -0.000000000000000000, 0.000000000000000000, -1.000000000000000000 ) ) ;
#23475=DIRECTION ( 'NONE',  ( 1.000000000000000000, -1.110223024625156540E-16, 0.000000000000000000 ) ) ;
#23485=PLANE ( 'NONE',  #12588 ) ;
#23500=DIRECTION ( 'NONE',  ( 0.000000000000000000, 0.000000000000000000, -1.000000000000000000 ) ) ;
#23512=DIRECTION ( 'NONE',  ( 0.000000000000000000, 0.000000000000000000, -1.000000000000000000 ) ) ;
#23521=DIRECTION ( 'NONE',  ( -0.000000000000000000, 0.000000000000000000, -1.000000000000000000 ) ) ;
#23524=EDGE_LOOP ( 'NONE', ( #34691, #6853, #30172, #6315, #35321 ) ) ;
#23568=CARTESIAN_POINT ( 'NONE',  ( -3.799999999999999822, 4.653657836759942730E-16, 60.00000000000000000 ) ) ;
#23576=DIRECTION ( 'NONE',  ( 0.000000000000000000, 0.000000000000000000, -1.000000000000000000 ) ) ;
#23619=CIRCLE ( 'NONE', #28218, 4.000000000000000000 ) ;
#23625=PRODUCT_DEFINITION_SHAPE ( 'NONE', 'NONE',  #6847 ) ;
#23644=EDGE_CURVE ( 'NONE', #17290, #18475, #17045, .T. ) ;
#23683=ADVANCED_FACE ( 'NONE', ( #30743 ), #3400, .T. ) ;
#23728=CARTESIAN_POINT ( 'NONE',  ( 3.799999999999999822, 0.000000000000000000, -44.50000000000000000 ) ) ;
#23736=CIRCLE ( 'NONE', #23159, 4.000000000000000000 ) ;
#23749=AXIS2_PLACEMENT_3D ( 'NONE', #27237, #13545, #5276 ) ;
#23773=ORIENTED_EDGE ( 'NONE', *, *, #26373, .T. ) ;
#23815=CYLINDRICAL_SURFACE ( 'NONE', #16445, 4.000000000000000000 ) ;
#23907=FACE_OUTER_BOUND ( 'NONE', #11284, .T. ) ;
#23911=CARTESIAN_POINT ( 'NONE',  ( 0.000000000000000000, 0.000000000000000000, 35.10000000000000142 ) ) ;
#23936=ORIENTED_EDGE ( 'NONE', *, *, #21841, .F. ) ;
#23956=ORIENTED_EDGE ( 'NONE', *, *, #7750, .F. ) ;
#24008=DIRECTION ( 'NONE',  ( 1.110223024625156540E-16, 1.000000000000000000, 0.000000000000000000 ) ) ;
#24013=FACE_BOUND ( 'NONE', #31751, .T. ) ;
#24042=DIRECTION ( 'NONE',  ( 0.000000000000000000, 0.000000000000000000, 1.000000000000000000 ) ) ;
#24056=ORIENTED_EDGE ( 'NONE', *, *, #31132, .F. ) ;
#24097=DIRECTION ( 'NONE',  ( 1.000000000000000000, 0.000000000000000000, 0.000000000000000000 ) ) ;
#24099=DIRECTION ( 'NONE',  ( -1.000000000000000000, 1.110223024625156540E-16, 0.000000000000000000 ) ) ;
#24112=ORIENTED_EDGE ( 'NONE', *, *, #16719, .T. ) ;
#24167=FACE_OUTER_BOUND ( 'NONE', #28610, .T. ) ;
#24190=DIRECTION ( 'NONE',  ( 0.000000000000000000, 1.000000000000000000, 0.000000000000000000 ) ) ;
#24231=CARTESIAN_POINT ( 'NONE',  ( 5.400000000000085620, -1.000000000000049516, -44.50000000000000000 ) ) ;
#24254=DIRECTION ( 'NONE',  ( 0.000000000000000000, 0.000000000000000000, -1.000000000000000000 ) ) ;
#24264=CIRCLE ( 'NONE', #28265, 4.000000000000000000 ) ;
#24330=CIRCLE ( 'NONE', #3048, 3.799999999999999822 ) ;
#24373=ORIENTED_EDGE ( 'NONE', *, *, #12808, .T. ) ;
#24424=DIRECTION ( 'NONE',  ( -0.000000000000000000, 0.000000000000000000, -1.000000000000000000 ) ) ;
#24437=DIRECTION ( 'NONE',  ( -0.000000000000000000, 0.000000000000000000, -1.000000000000000000 ) ) ;
#24456=AXIS2_PLACEMENT_3D ( 'NONE', #32360, #5362, #26437 ) ;
#24483=FACE_OUTER_BOUND ( 'NONE', #11729, .T. ) ;
#24508=VERTEX_POINT ( 'NONE', #15508 ) ;
#24555=EDGE_LOOP ( 'NONE', ( #11914, #31367 ) ) ;
#24606=DIRECTION ( 'NONE',  ( 0.000000000000000000, 0.000000000000000000, 1.000000000000000000 ) ) ;
#24616=DIRECTION ( 'NONE',  ( 1.000000000000000000, 0.000000000000000000, 0.000000000000000000 ) ) ;
#24628=LINE ( 'NONE', #32903, #20506 ) ;
#24642=DIRECTION ( 'NONE',  ( -1.000000000000000000, 0.000000000000000000, 0.000000000000000000 ) ) ;
#24673=EDGE_CURVE ( 'NONE', #31584, #1546, #13526, .T. ) ;
#24705=ORIENTED_EDGE ( 'NONE', *, *, #18970, .T. ) ;
#24724=ORIENTED_EDGE ( 'NONE', *, *, #29694, .T. ) ;
#24746=ADVANCED_FACE ( 'NONE', ( #3805 ), #25770, .T. ) ;
#24837=ORIENTED_EDGE ( 'NONE', *, *, #23644, .F. ) ;
#24848=AXIS2_PLACEMENT_3D ( 'NONE', #10209, #4465, #15944 ) ;
#24901=DIRECTION ( 'NONE',  ( -1.000000000000000000, 0.000000000000000000, 0.000000000000000000 ) ) ;
#24915=CARTESIAN_POINT ( 'NONE',  ( 5.400000000000071410, 0.9999999999999662492, 55.00000000000000711 ) ) ;
#24933=DIRECTION ( 'NONE',  ( 0.000000000000000000, 0.000000000000000000, -1.000000000000000000 ) ) ;
#24970=AXIS2_PLACEMENT_3D ( 'NONE', #34411, #17995, #6487 ) ;
#24997=CYLINDRICAL_SURFACE ( 'NONE', #26445, 3.799999999999999822 ) ;
#25153=ADVANCED_FACE ( 'NONE', ( #24483 ), #30238, .T. ) ;
#25158=DIRECTION ( 'NONE',  ( -1.000000000000000000, 0.000000000000000000, 0.000000000000000000 ) ) ;
#25160=ORIENTED_EDGE ( 'NONE', *, *, #30560, .T. ) ;
#25179=DIRECTION ( 'NONE',  ( 0.000000000000000000, 0.000000000000000000, 1.000000000000000000 ) ) ;
#25199=ORIENTED_EDGE ( 'NONE', *, *, #313, .F. ) ;
#25207=CARTESIAN_POINT ( 'NONE',  ( 5.400000000000085620, -1.000000000000049516, 53.00000000000000711 ) ) ;
#25232=DIRECTION ( 'NONE',  ( -1.000000000000000000, 0.000000000000000000, 0.000000000000000000 ) ) ;
#25258=ORIENTED_EDGE ( 'NONE', *, *, #26434, .T. ) ;
#25365=EDGE_CURVE ( 'NONE', #5282, #34581, #14530, .T. ) ;
#25420=ORIENTED_EDGE ( 'NONE', *, *, #8591, .F. ) ;
#25484=CIRCLE ( 'NONE', #3086, 3.799999999999999822 ) ;
#25519=DIRECTION ( 'NONE',  ( 0.000000000000000000, 0.000000000000000000, 1.000000000000000000 ) ) ;
#25542=DIRECTION ( 'NONE',  ( 1.000000000000000000, 0.000000000000000000, 0.000000000000000000 ) ) ;
#25566=ORIENTED_EDGE ( 'NONE', *, *, #35060, .F. ) ;
#25567=EDGE_CURVE ( 'NONE', #35528, #708, #21365, .T. ) ;
#25604=EDGE_CURVE ( 'NONE', #1850, #2693, #5361, .T. ) ;
#25621=ORIENTED_EDGE ( 'NONE', *, *, #29094, .F. ) ;
#25637=CARTESIAN_POINT ( 'NONE',  ( 3.799999999999999822, 0.000000000000000000, 60.00000000000000000 ) ) ;
#25738=EDGE_LOOP ( 'NONE', ( #33747, #29287 ) ) ;
#25739=ORIENTED_EDGE ( 'NONE', *, *, #20745, .F. ) ;
#25770=CYLINDRICAL_SURFACE ( 'NONE', #6063, 4.000000000000000000 ) ;
#25822=CARTESIAN_POINT ( 'NONE',  ( 0.000000000000000000, 0.000000000000000000, -32.00000000000000000 ) ) ;
#25859=CIRCLE ( 'NONE', #3431, 4.000000000000000000 ) ;
#25920=CARTESIAN_POINT ( 'NONE',  ( 1.110223024625156540E-13, -1.000000000000042633, 45.00000000000000711 ) ) ;
#25967=ORIENTED_EDGE ( 'NONE', *, *, #759, .F. ) ;
#26007=CIRCLE ( 'NONE', #31163, 3.799999999999999822 ) ;
#26077=DIRECTION ( 'NONE',  ( 0.000000000000000000, 0.000000000000000000, -1.000000000000000000 ) ) ;
#26080=CARTESIAN_POINT ( 'NONE',  ( 0.000000000000000000, 0.000000000000000000, -40.00000000000000000 ) ) ;
#26099=ORIENTED_EDGE ( 'NONE', *, *, #5616, .F. ) ;
#26130=DIRECTION ( 'NONE',  ( -1.000000000000000000, 0.000000000000000000, 0.000000000000000000 ) ) ;
#26146=VERTEX_POINT ( 'NONE', #29984 ) ;
#26155=CARTESIAN_POINT ( 'NONE',  ( 0.000000000000000000, 0.000000000000000000, -52.50000000000000000 ) ) ;
#26159=CARTESIAN_POINT ( 'NONE',  ( 0.000000000000000000, 0.000000000000000000, -52.50000000000000000 ) ) ;
#26170=DIRECTION ( 'NONE',  ( -1.000000000000000000, 0.000000000000000000, 0.000000000000000000 ) ) ;
#26221=ORIENTED_EDGE ( 'NONE', *, *, #30560, .F. ) ;
#26266=CARTESIAN_POINT ( 'NONE',  ( 5.400000000000071410, 0.9999999999999662492, 55.00000000000000711 ) ) ;
#26350=LINE ( 'NONE', #23268, #17982 ) ;
#26352=DIRECTION ( 'NONE',  ( 0.000000000000000000, 0.000000000000000000, 1.000000000000000000 ) ) ;
#26373=EDGE_CURVE ( 'NONE', #3282, #17290, #24330, .T. ) ;
#26388=ORIENTED_EDGE ( 'NONE', *, *, #25567, .T. ) ;
#26401=FILL_AREA_STYLE ('',( #34685 ) ) ;
#26416=CIRCLE ( 'NONE', #27047, 4.000000000000000000 ) ;
#26434=EDGE_CURVE ( 'NONE', #15509, #19295, #14627, .T. ) ;
#26437=DIRECTION ( 'NONE',  ( -1.000000000000000000, 0.000000000000000000, 0.000000000000000000 ) ) ;
#26445=AXIS2_PLACEMENT_3D ( 'NONE', #21931, #19408, #19912 ) ;
#26480=DIRECTION ( 'NONE',  ( 0.000000000000000000, 0.000000000000000000, -1.000000000000000000 ) ) ;
#26496=DIRECTION ( 'NONE',  ( 0.000000000000000000, 0.000000000000000000, -1.000000000000000000 ) ) ;
#26510=( LENGTH_UNIT ( ) NAMED_UNIT ( * ) SI_UNIT ( .MILLI., .METRE. ) );
#26529=ORIENTED_EDGE ( 'NONE', *, *, #6968, .T. ) ;
#26556=( GEOMETRIC_REPRESENTATION_CONTEXT ( 3 ) GLOBAL_UNCERTAINTY_ASSIGNED_CONTEXT ( ( #19716 ) ) GLOBAL_UNIT_ASSIGNED_CONTEXT ( ( #26510, #29565, #1844 ) ) REPRESENTATION_CONTEXT ( 'NONE', 'WORKASPACE' ) );
#26589=CARTESIAN_POINT ( 'NONE',  ( 0.000000000000000000, 0.000000000000000000, 0.000000000000000000 ) ) ;
#26617=DIRECTION ( 'NONE',  ( 1.000000000000000000, 0.000000000000000000, 0.000000000000000000 ) ) ;
#26634=ORIENTED_EDGE ( 'NONE', *, *, #27732, .T. ) ;
#26653=VECTOR ( 'NONE', #27671, 1000.000000000000000 ) ;
#26664=DIRECTION ( 'NONE',  ( 0.000000000000000000, 0.000000000000000000, 1.000000000000000000 ) ) ;
#26751=EDGE_LOOP ( 'NONE', ( #26221, #12988 ) ) ;
#26777=VECTOR ( 'NONE', #14821, 1000.000000000000000 ) ;
#26806=EDGE_LOOP ( 'NONE', ( #31254, #22917, #13409, #29519 ) ) ;
#26863=SURFACE_STYLE_USAGE ( .BOTH. , #4898 ) ;
#26870=VECTOR ( 'NONE', #12178, 1000.000000000000000 ) ;
#26902=DIRECTION ( 'NONE',  ( -1.000000000000000000, 0.000000000000000000, 0.000000000000000000 ) ) ;
#26904=LINE ( 'NONE', #18598, #946 ) ;
#26930=ORIENTED_EDGE ( 'NONE', *, *, #14825, .T. ) ;
#26989=ORIENTED_EDGE ( 'NONE', *, *, #32627, .F. ) ;
#27011=DIRECTION ( 'NONE',  ( 0.000000000000000000, 0.000000000000000000, 1.000000000000000000 ) ) ;
#27026=ORIENTED_EDGE ( 'NONE', *, *, #14825, .F. ) ;
#27029=LINE ( 'NONE', #10461, #22626 ) ;
#27039=FILL_AREA_STYLE ('',( #15667 ) ) ;
#27043=CIRCLE ( 'NONE', #22404, 3.799999999999999822 ) ;
#27047=AXIS2_PLACEMENT_3D ( 'NONE', #17851, #31896, #23450 ) ;
#27048=ORIENTED_EDGE ( 'NONE', *, *, #16775, .T. ) ;
#27058=ORIENTED_EDGE ( 'NONE', *, *, #31259, .F. ) ;
#27087=DIRECTION ( 'NONE',  ( 0.000000000000000000, 0.000000000000000000, -1.000000000000000000 ) ) ;
#27091=CYLINDRICAL_SURFACE ( 'NONE', #14384, 4.000000000000000000 ) ;
#27098=FACE_OUTER_BOUND ( 'NONE', #9933, .T. ) ;
#27106=ORIENTED_EDGE ( 'NONE', *, *, #14000, .F. ) ;
#27110=LINE ( 'NONE', #21866, #19554 ) ;
#27113=DIRECTION ( 'NONE',  ( 0.000000000000000000, 1.000000000000000000, 0.000000000000000000 ) ) ;
#27218=ORIENTED_EDGE ( 'NONE', *, *, #28894, .F. ) ;
#27232=VECTOR ( 'NONE', #25179, 1000.000000000000000 ) ;
#27237=CARTESIAN_POINT ( 'NONE',  ( 0.000000000000000000, 0.000000000000000000, -65.00000000000000000 ) ) ;
#27289=ORIENTED_EDGE ( 'NONE', *, *, #22461, .F. ) ;
#27290=VECTOR ( 'NONE', #7693, 1000.000000000000000 ) ;
#27314=LINE ( 'NONE', #8212, #26653 ) ;
#27337=CLOSED_SHELL ( 'NONE', ( #29307, #31936, #5559, #33201, #13203, #18552, #9083, #13305, #4069, #23683, #25153, #2286, #30156, #21076, #3328, #20046, #15201, #17358, #18555, #4852, #8391, #16806, #21683, #21168, #6520, #1386, #5695, #3818, #1792, #4736, #18649, #5108, #21886, #6589, #1627, #14040, #10642, #16066, #28235, #926, #14791, #10382, #681, #24746, #4884, #32591, #17579, #13530, #11520, #9036, #16650, #20202, #19546, #14039, #33713, #12103, #19211 ) ) ;
#27347=EDGE_CURVE ( 'NONE', #15054, #2693, #11805, .T. ) ;
#27351=ORIENTED_EDGE ( 'NONE', *, *, #33890, .F. ) ;
#27352=CARTESIAN_POINT ( 'NONE',  ( -4.000000000000000000, 0.000000000000000000, -31.10000000000000142 ) ) ;
#27445=CYLINDRICAL_SURFACE ( 'NONE', #9131, 4.000000000000000000 ) ;
#27478=CARTESIAN_POINT ( 'NONE',  ( 0.000000000000000000, 0.000000000000000000, 65.00000000000000000 ) ) ;
#27570=EDGE_LOOP ( 'NONE', ( #33348, #18672, #6946, #22602 ) ) ;
#27574=DIRECTION ( 'NONE',  ( 1.000000000000000000, 0.000000000000000000, 0.000000000000000000 ) ) ;
#27594=CARTESIAN_POINT ( 'NONE',  ( 0.000000000000000000, 0.000000000000000000, -43.60000000000000142 ) ) ;
#27625=DIRECTION ( 'NONE',  ( -1.000000000000000000, 0.000000000000000000, 0.000000000000000000 ) ) ;
#27629=CARTESIAN_POINT ( 'NONE',  ( -4.000000000000000000, 0.000000000000000000, -52.50000000000000000 ) ) ;
#27652=CARTESIAN_POINT ( 'NONE',  ( -4.000000000000000000, 0.000000000000000000, -65.00000000000000000 ) ) ;
#27671=DIRECTION ( 'NONE',  ( 1.000000000000000000, 5.551115123125782702E-16, 0.000000000000000000 ) ) ;
#27697=CARTESIAN_POINT ( 'NONE',  ( 3.799999999999999822, 0.000000000000000000, -44.50000000000000000 ) ) ;
#27706=ORIENTED_EDGE ( 'NONE', *, *, #17350, .T. ) ;
#27732=EDGE_CURVE ( 'NONE', #18475, #35360, #29061, .T. ) ;
#27762=EDGE_CURVE ( 'NONE', #33416, #2210, #18119, .T. ) ;
#27768=CIRCLE ( 'NONE', #23749, 4.000000000000000000 ) ;
#27788=CARTESIAN_POINT ( 'NONE',  ( 0.000000000000000000, 0.000000000000000000, -31.10000000000000142 ) ) ;
#27815=DIRECTION ( 'NONE',  ( -0.000000000000000000, 0.000000000000000000, -1.000000000000000000 ) ) ;
#27823=LINE ( 'NONE', #16641, #16537 ) ;
#27833=EDGE_CURVE ( 'NONE', #15509, #9289, #13562, .T. ) ;
#27907=DIRECTION ( 'NONE',  ( -0.000000000000000000, 0.000000000000000000, -1.000000000000000000 ) ) ;
#27940=CARTESIAN_POINT ( 'NONE',  ( 5.400000000000085620, -1.000000000000049516, -32.00000000000000000 ) ) ;
#27946=ORIENTED_EDGE ( 'NONE', *, *, #9445, .T. ) ;
#27954=CIRCLE ( 'NONE', #34278, 4.000000000000000000 ) ;
#27969=VECTOR ( 'NONE', #29703, 1000.000000000000000 ) ;
#27970=DIRECTION ( 'NONE',  ( 0.000000000000000000, 0.000000000000000000, -1.000000000000000000 ) ) ;
#27992=CARTESIAN_POINT ( 'NONE',  ( 0.000000000000000000, 0.000000000000000000, -52.50000000000000000 ) ) ;
#27999=CIRCLE ( 'NONE', #5004, 4.000000000000000000 ) ;
#28000=EDGE_LOOP ( 'NONE', ( #25199, #13300 ) ) ;
#28028=DIRECTION ( 'NONE',  ( -1.000000000000000000, 0.000000000000000000, 0.000000000000000000 ) ) ;
#28041=LINE ( 'NONE', #16678, #12568 ) ;
#28048=FACE_OUTER_BOUND ( 'NONE', #17202, .T. ) ;
#28077=EDGE_LOOP ( 'NONE', ( #15004, #12037, #16197, #24837 ) ) ;
#28098=DIRECTION ( 'NONE',  ( -1.000000000000000000, 0.000000000000000000, 0.000000000000000000 ) ) ;
#28102=CARTESIAN_POINT ( 'NONE',  ( -3.799999999999999822, 4.653657836759942730E-16, -40.89999999999999858 ) ) ;
#28110=AXIS2_PLACEMENT_3D ( 'NONE', #35195, #27087, #27625 ) ;
#28136=EDGE_LOOP ( 'NONE', ( #12350, #16216 ) ) ;
#28168=VERTEX_POINT ( 'NONE', #1062 ) ;
#28200=DIRECTION ( 'NONE',  ( 0.000000000000000000, 0.000000000000000000, -1.000000000000000000 ) ) ;
#28208=CARTESIAN_POINT ( 'NONE',  ( 5.400000000000085620, -1.000000000000049516, 45.00000000000000711 ) ) ;
#28217=CIRCLE ( 'NONE', #10950, 3.799999999999999822 ) ;
#28218=AXIS2_PLACEMENT_3D ( 'NONE', #5604, #27907, #27574 ) ;
#28220=LINE ( 'NONE', #3558, #22720 ) ;
#28221=DIRECTION ( 'NONE',  ( 1.000000000000000000, 0.000000000000000000, 0.000000000000000000 ) ) ;
#28235=ADVANCED_FACE ( 'NONE', ( #14535, #4129 ), #6804, .F. ) ;
#28259=DIRECTION ( 'NONE',  ( -1.000000000000000000, 0.000000000000000000, 0.000000000000000000 ) ) ;
#28265=AXIS2_PLACEMENT_3D ( 'NONE', #30919, #19906, #24642 ) ;
#28355=EDGE_CURVE ( 'NONE', #15935, #31584, #7158, .T. ) ;
#28362=DIRECTION ( 'NONE',  ( -0.000000000000000000, 0.000000000000000000, -1.000000000000000000 ) ) ;
#28390=CYLINDRICAL_SURFACE ( 'NONE', #18122, 3.799999999999999822 ) ;
#28415=EDGE_CURVE ( 'NONE', #14157, #18547, #8410, .T. ) ;
#28425=ORIENTED_EDGE ( 'NONE', *, *, #12873, .T. ) ;
#28451=DIRECTION ( 'NONE',  ( -1.000000000000000000, 0.000000000000000000, 0.000000000000000000 ) ) ;
#28476=EDGE_CURVE ( 'NONE', #5329, #14055, #16446, .T. ) ;
#28481=DIRECTION ( 'NONE',  ( -1.000000000000000000, 0.000000000000000000, 0.000000000000000000 ) ) ;
#28516=EDGE_LOOP ( 'NONE', ( #32575, #6550, #32152, #21854 ) ) ;
#28529=ORIENTED_EDGE ( 'NONE', *, *, #29628, .F. ) ;
#28610=EDGE_LOOP ( 'NONE', ( #11355, #32368, #19255, #13633, #24056, #21297, #31579, #7559 ) ) ;
#28612=DIRECTION ( 'NONE',  ( 0.000000000000000000, 0.000000000000000000, -1.000000000000000000 ) ) ;
#28624=CIRCLE ( 'NONE', #2793, 4.000000000000000000 ) ;
#28645=DIRECTION ( 'NONE',  ( -0.000000000000000000, 0.000000000000000000, -1.000000000000000000 ) ) ;
#28681=VECTOR ( 'NONE', #15358, 1000.000000000000000 ) ;
#28742=CARTESIAN_POINT ( 'NONE',  ( 3.799999999999999822, 0.000000000000000000, -40.89999999999999858 ) ) ;
#28772=CARTESIAN_POINT ( 'NONE',  ( 4.000000000000000000, 4.898587196589412829E-16, 65.00000000000000000 ) ) ;
#28801=CARTESIAN_POINT ( 'NONE',  ( 0.000000000000000000, 0.000000000000000000, 35.10000000000000142 ) ) ;
#28820=VERTEX_POINT ( 'NONE', #14859 ) ;
#28848=DIRECTION ( 'NONE',  ( -0.000000000000000000, 0.000000000000000000, -1.000000000000000000 ) ) ;
#28884=VERTEX_POINT ( 'NONE', #15198 ) ;
#28885=VERTEX_POINT ( 'NONE', #35047 ) ;
#28894=EDGE_CURVE ( 'NONE', #19681, #17706, #4439, .T. ) ;
#28906=FACE_OUTER_BOUND ( 'NONE', #20755, .T. ) ;
#28921=DIRECTION ( 'NONE',  ( -0.000000000000000000, 0.000000000000000000, -1.000000000000000000 ) ) ;
#28946=CYLINDRICAL_SURFACE ( 'NONE', #9981, 3.799999999999999822 ) ;
#28948=CARTESIAN_POINT ( 'NONE',  ( 3.799999999999999822, 0.000000000000000000, -32.00000000000000000 ) ) ;
#28952=AXIS2_PLACEMENT_3D ( 'NONE', #559, #6317, #2935 ) ;
#28967=VERTEX_POINT ( 'NONE', #18630 ) ;
#28975=ORIENTED_EDGE ( 'NONE', *, *, #5738, .F. ) ;
#28981=EDGE_LOOP ( 'NONE', ( #8739, #14429, #34919, #8125, #34777 ) ) ;
#28988=CARTESIAN_POINT ( 'NONE',  ( 0.000000000000000000, 0.000000000000000000, -55.89999999999999858 ) ) ;
#29029=AXIS2_PLACEMENT_3D ( 'NONE', #23911, #21529, #26617 ) ;
#29034=LINE ( 'NONE', #6525, #7816 ) ;
#29039=DIRECTION ( 'NONE',  ( 1.000000000000000000, 0.000000000000000000, 0.000000000000000000 ) ) ;
#29051=LINE ( 'NONE', #12854, #17607 ) ;
#29061=CIRCLE ( 'NONE', #11795, 3.799999999999999822 ) ;
#29081=CARTESIAN_POINT ( 'NONE',  ( -3.799999999999999822, 4.653657836759942730E-16, -44.50000000000000000 ) ) ;
#29094=EDGE_CURVE ( 'NONE', #10066, #13424, #21865, .T. ) ;
#29122=ORIENTED_EDGE ( 'NONE', *, *, #5407, .F. ) ;
#29145=AXIS2_PLACEMENT_3D ( 'NONE', #4666, #29851, #18318 ) ;
#29156=AXIS2_PLACEMENT_3D ( 'NONE', #21464, #10141, #18417 ) ;
#29171=DIRECTION ( 'NONE',  ( 1.000000000000000000, 0.000000000000000000, 0.000000000000000000 ) ) ;
#29177=CARTESIAN_POINT ( 'NONE',  ( 0.000000000000000000, 0.000000000000000000, 35.10000000000000142 ) ) ;
#29234=LINE ( 'NONE', #20567, #22604 ) ;
#29287=ORIENTED_EDGE ( 'NONE', *, *, #17852, .T. ) ;
#29291=EDGE_LOOP ( 'NONE', ( #12790, #13199, #22039, #7375 ) ) ;
#29307=ADVANCED_FACE ( 'NONE', ( #32072 ), #21252, .T. ) ;
#29316=DIRECTION ( 'NONE',  ( 0.000000000000000000, 0.000000000000000000, -1.000000000000000000 ) ) ;
#29341=VERTEX_POINT ( 'NONE', #21596 ) ;
#29344=CARTESIAN_POINT ( 'NONE',  ( 5.400000000000071410, 0.9999999999999662492, -32.00000000000000000 ) ) ;
#29384=SURFACE_STYLE_FILL_AREA ( #27039 ) ;
#29389=ORIENTED_EDGE ( 'NONE', *, *, #34791, .T. ) ;
#29402=DIRECTION ( 'NONE',  ( -1.000000000000000000, 0.000000000000000000, 0.000000000000000000 ) ) ;
#29412=DIRECTION ( 'NONE',  ( -1.000000000000000000, 0.000000000000000000, 0.000000000000000000 ) ) ;
#29445=DIRECTION ( 'NONE',  ( -1.000000000000000000, 0.000000000000000000, 0.000000000000000000 ) ) ;
#29500=CARTESIAN_POINT ( 'NONE',  ( 3.872983346207517386, -1.000000000000028644, 65.00000000000000000 ) ) ;
#29519=ORIENTED_EDGE ( 'NONE', *, *, #8411, .T. ) ;
#29553=DIRECTION ( 'NONE',  ( 0.000000000000000000, 0.000000000000000000, 1.000000000000000000 ) ) ;
#29565=( NAMED_UNIT ( * ) PLANE_ANGLE_UNIT ( ) SI_UNIT ( $, .RADIAN. ) );
#29582=VECTOR ( 'NONE', #35271, 1000.000000000000000 ) ;
#29590=EDGE_CURVE ( 'NONE', #32739, #15054, #31135, .T. ) ;
#29628=EDGE_CURVE ( 'NONE', #35092, #11309, #11938, .T. ) ;
#29633=LINE ( 'NONE', #24231, #22269 ) ;
#29635=ORIENTED_EDGE ( 'NONE', *, *, #1104, .F. ) ;
#29694=EDGE_CURVE ( 'NONE', #33209, #17384, #28624, .T. ) ;
#29703=DIRECTION ( 'NONE',  ( -0.000000000000000000, 0.000000000000000000, -1.000000000000000000 ) ) ;
#29716=EDGE_LOOP ( 'NONE', ( #33895, #24112, #5985, #15128 ) ) ;
#29742=STYLED_ITEM ( 'NONE', ( #9298 ), #34226 ) ;
#29747=EDGE_CURVE ( 'NONE', #24508, #31889, #12533, .T. ) ;
#29788=CIRCLE ( 'NONE', #7276, 3.799999999999999822 ) ;
#29793=CARTESIAN_POINT ( 'NONE',  ( -4.000000000000000000, 0.000000000000000000, 60.90000000000001279 ) ) ;
#29851=DIRECTION ( 'NONE',  ( 0.000000000000000000, 0.000000000000000000, -1.000000000000000000 ) ) ;
#29858=EDGE_LOOP ( 'NONE', ( #31552, #30483, #22488, #14678 ) ) ;
#29871=ORIENTED_EDGE ( 'NONE', *, *, #8821, .T. ) ;
#29889=CIRCLE ( 'NONE', #5175, 3.799999999999999822 ) ;
#29911=( LENGTH_UNIT ( ) NAMED_UNIT ( * ) SI_UNIT ( .MILLI., .METRE. ) );
#29912=CARTESIAN_POINT ( 'NONE',  ( 5.400000000000085620, -1.000000000000049516, -40.00000000000000000 ) ) ;
#29966=DIRECTION ( 'NONE',  ( -0.000000000000000000, 0.000000000000000000, -1.000000000000000000 ) ) ;
#29984=CARTESIAN_POINT ( 'NONE',  ( 4.000000000000000000, 4.898587196589412829E-16, 35.10000000000000142 ) ) ;
#30006=DIRECTION ( 'NONE',  ( 1.000000000000000000, 0.000000000000000000, 0.000000000000000000 ) ) ;
#30072=ORIENTED_EDGE ( 'NONE', *, *, #9901, .T. ) ;
#30098=CARTESIAN_POINT ( 'NONE',  ( -3.799999999999999822, 4.653657836759942730E-16, -55.89999999999999858 ) ) ;
#30123=EDGE_LOOP ( 'NONE', ( #27351, #26989 ) ) ;
#30126=EDGE_CURVE ( 'NONE', #18547, #34626, #28220, .T. ) ;
#30130=ORIENTED_EDGE ( 'NONE', *, *, #15823, .F. ) ;
#30134=CARTESIAN_POINT ( 'NONE',  ( 0.000000000000000000, 0.000000000000000000, 36.00000000000000000 ) ) ;
#30138=DIRECTION ( 'NONE',  ( -1.000000000000000000, 0.000000000000000000, 0.000000000000000000 ) ) ;
#30156=ADVANCED_FACE ( 'NONE', ( #15530 ), #28390, .T. ) ;
#30172=ORIENTED_EDGE ( 'NONE', *, *, #34838, .T. ) ;
#30187=VECTOR ( 'NONE', #15242, 1000.000000000000000 ) ;
#30238=CYLINDRICAL_SURFACE ( 'NONE', #2665, 3.799999999999999822 ) ;
#30256=VECTOR ( 'NONE', #6444, 1000.000000000000000 ) ;
#30269=ORIENTED_EDGE ( 'NONE', *, *, #14284, .T. ) ;
#30291=CIRCLE ( 'NONE', #21627, 4.000000000000000000 ) ;
#30322=LINE ( 'NONE', #24915, #4477 ) ;
#30326=FACE_OUTER_BOUND ( 'NONE', #28136, .T. ) ;
#30333=EDGE_CURVE ( 'NONE', #10690, #15000, #21469, .T. ) ;
#30355=AXIS2_PLACEMENT_3D ( 'NONE', #1425, #17255, #28259 ) ;
#30387=PLANE ( 'NONE',  #31392 ) ;
#30452=ORIENTED_EDGE ( 'NONE', *, *, #313, .T. ) ;
#30457=DIRECTION ( 'NONE',  ( 0.000000000000000000, 0.000000000000000000, -1.000000000000000000 ) ) ;
#30483=ORIENTED_EDGE ( 'NONE', *, *, #4281, .F. ) ;
#30549=CIRCLE ( 'NONE', #16732, 4.000000000000000000 ) ;
#30552=FACE_OUTER_BOUND ( 'NONE', #29858, .T. ) ;
#30557=DIRECTION ( 'NONE',  ( 1.000000000000000000, -1.110223024625156540E-16, 0.000000000000000000 ) ) ;
#30560=EDGE_CURVE ( 'NONE', #12699, #708, #3777, .T. ) ;
#30571=STYLED_ITEM ( 'NONE', ( #4558 ), #13375 ) ;
#30578=CARTESIAN_POINT ( 'NONE',  ( 4.000000000000000000, 4.898587196589412829E-16, -43.60000000000000142 ) ) ;
#30580=DIRECTION ( 'NONE',  ( 0.000000000000000000, 0.000000000000000000, -1.000000000000000000 ) ) ;
#30587=ORIENTED_EDGE ( 'NONE', *, *, #18138, .F. ) ;
#30607=EDGE_CURVE ( 'NONE', #19681, #529, #10952, .T. ) ;
#30619=FACE_OUTER_BOUND ( 'NONE', #29716, .T. ) ;
#30701=ORIENTED_EDGE ( 'NONE', *, *, #32128, .T. ) ;
#30737=PRODUCT_CONTEXT ( 'NONE', #35176, 'mechanical' ) ;
#30743=FACE_OUTER_BOUND ( 'NONE', #31339, .T. ) ;
#30778=ORIENTED_EDGE ( 'NONE', *, *, #16872, .T. ) ;
#30804=DIRECTION ( 'NONE',  ( 0.000000000000000000, 0.000000000000000000, -1.000000000000000000 ) ) ;
#30823=AXIS2_PLACEMENT_3D ( 'NONE', #16038, #13540, #29402 ) ;
#30856=CARTESIAN_POINT ( 'NONE',  ( 0.000000000000000000, 0.000000000000000000, -44.50000000000000000 ) ) ;
#30866=DIRECTION ( 'NONE',  ( -1.000000000000000000, 0.000000000000000000, 0.000000000000000000 ) ) ;
#30868=ORIENTED_EDGE ( 'NONE', *, *, #30607, .F. ) ;
#30905=VERTEX_POINT ( 'NONE', #29912 ) ;
#30919=CARTESIAN_POINT ( 'NONE',  ( 0.000000000000000000, 0.000000000000000000, 36.00000000000000000 ) ) ;
#30940=EDGE_LOOP ( 'NONE', ( #4366, #29871, #5371, #21253 ) ) ;
#30949=DIRECTION ( 'NONE',  ( 1.000000000000000000, 0.000000000000000000, 0.000000000000000000 ) ) ;
#30967=EDGE_LOOP ( 'NONE', ( #13141, #9647, #6577, #6473, #7359 ) ) ;
#31000=CYLINDRICAL_SURFACE ( 'NONE', #19354, 4.000000000000000000 ) ;
#31029=CARTESIAN_POINT ( 'NONE',  ( 3.799999999999999822, 0.000000000000000000, -53.39999999999999858 ) ) ;
#31038=ORIENTED_EDGE ( 'NONE', *, *, #1997, .T. ) ;
#31053=EDGE_CURVE ( 'NONE', #10066, #35092, #23619, .T. ) ;
#31064=FACE_OUTER_BOUND ( 'NONE', #10629, .T. ) ;
#31077=DIRECTION ( 'NONE',  ( 0.000000000000000000, 0.000000000000000000, -1.000000000000000000 ) ) ;
#31078=ORIENTED_EDGE ( 'NONE', *, *, #14688, .T. ) ;
#31105=CARTESIAN_POINT ( 'NONE',  ( -4.000000000000000000, 0.000000000000000000, -44.50000000000000000 ) ) ;
#31132=EDGE_CURVE ( 'NONE', #28967, #13424, #5277, .T. ) ;
#31135=LINE ( 'NONE', #25920, #3912 ) ;
#31149=DIRECTION ( 'NONE',  ( -1.000000000000000000, 0.000000000000000000, 0.000000000000000000 ) ) ;
#31163=AXIS2_PLACEMENT_3D ( 'NONE', #6387, #22940, #19864 ) ;
#31179=DIRECTION ( 'NONE',  ( -0.000000000000000000, 0.000000000000000000, -1.000000000000000000 ) ) ;
#31204=DIRECTION ( 'NONE',  ( 0.000000000000000000, 0.000000000000000000, 1.000000000000000000 ) ) ;
#31244=EDGE_CURVE ( 'NONE', #1732, #19003, #30549, .T. ) ;
#31254=ORIENTED_EDGE ( 'NONE', *, *, #2012, .F. ) ;
#31259=EDGE_CURVE ( 'NONE', #9289, #11649, #15266, .T. ) ;
#31261=EDGE_LOOP ( 'NONE', ( #33006, #27289, #14301, #25160 ) ) ;
#31286=AXIS2_PLACEMENT_3D ( 'NONE', #9897, #23414, #15109 ) ;
#31303=ORIENTED_EDGE ( 'NONE', *, *, #22089, .F. ) ;
#31305=CARTESIAN_POINT ( 'NONE',  ( 5.400000000000071410, 0.9999999999999662492, -44.50000000000000000 ) ) ;
#31309=DIRECTION ( 'NONE',  ( -1.000000000000000000, 0.000000000000000000, 0.000000000000000000 ) ) ;
#31321=EDGE_CURVE ( 'NONE', #14882, #2210, #4853, .T. ) ;
#31339=EDGE_LOOP ( 'NONE', ( #31683, #1131, #8418, #30587 ) ) ;
#31345=DIRECTION ( 'NONE',  ( 0.000000000000000000, 0.000000000000000000, -1.000000000000000000 ) ) ;
#31367=ORIENTED_EDGE ( 'NONE', *, *, #21969, .T. ) ;
#31377=DIRECTION ( 'NONE',  ( -0.000000000000000000, 0.000000000000000000, -1.000000000000000000 ) ) ;
#31392=AXIS2_PLACEMENT_3D ( 'NONE', #3549, #25158, #6061 ) ;
#31406=FACE_OUTER_BOUND ( 'NONE', #32906, .T. ) ;
#31410=FACE_OUTER_BOUND ( 'NONE', #34043, .T. ) ;
#31448=CIRCLE ( 'NONE', #23400, 4.000000000000000000 ) ;
#31497=DIRECTION ( 'NONE',  ( 1.000000000000000000, -1.110223024625156540E-16, 0.000000000000000000 ) ) ;
#31515=CARTESIAN_POINT ( 'NONE',  ( 0.000000000000000000, 0.000000000000000000, 45.00000000000000711 ) ) ;
#31532=CARTESIAN_POINT ( 'NONE',  ( 0.000000000000000000, 0.000000000000000000, 60.90000000000001279 ) ) ;
#31552=ORIENTED_EDGE ( 'NONE', *, *, #8364, .F. ) ;
#31565=DIRECTION ( 'NONE',  ( 0.000000000000000000, 0.000000000000000000, -1.000000000000000000 ) ) ;
#31569=EDGE_CURVE ( 'NONE', #8675, #28820, #24264, .T. ) ;
#31579=ORIENTED_EDGE ( 'NONE', *, *, #31569, .F. ) ;
#31584=VERTEX_POINT ( 'NONE', #1570 ) ;
#31663=CARTESIAN_POINT ( 'NONE',  ( 0.000000000000000000, 0.000000000000000000, 45.00000000000000711 ) ) ;
#31683=ORIENTED_EDGE ( 'NONE', *, *, #11069, .T. ) ;
#31702=EDGE_LOOP ( 'NONE', ( #27026, #30072, #30701, #15427 ) ) ;
#31725=( GEOMETRIC_REPRESENTATION_CONTEXT ( 3 ) GLOBAL_UNCERTAINTY_ASSIGNED_CONTEXT ( ( #6065 ) ) GLOBAL_UNIT_ASSIGNED_CONTEXT ( ( #29911, #10296, #34781 ) ) REPRESENTATION_CONTEXT ( 'NONE', 'WORKASPACE' ) );
#31744=CYLINDRICAL_SURFACE ( 'NONE', #11327, 4.000000000000000000 ) ;
#31751=EDGE_LOOP ( 'NONE', ( #18372, #2537 ) ) ;
#31765=CYLINDRICAL_SURFACE ( 'NONE', #18403, 4.000000000000000000 ) ;
#31780=DIRECTION ( 'NONE',  ( 0.000000000000000000, 0.000000000000000000, -1.000000000000000000 ) ) ;
#31797=VERTEX_POINT ( 'NONE', #7665 ) ;
#31817=CARTESIAN_POINT ( 'NONE',  ( 0.000000000000000000, 0.000000000000000000, 60.00000000000000000 ) ) ;
#31830=ORIENTED_EDGE ( 'NONE', *, *, #6419, .F. ) ;
#31852=DIRECTION ( 'NONE',  ( 0.000000000000000000, 0.000000000000000000, 1.000000000000000000 ) ) ;
#31889=VERTEX_POINT ( 'NONE', #21175 ) ;
#31891=EDGE_CURVE ( 'NONE', #9483, #7515, #9316, .T. ) ;
#31896=DIRECTION ( 'NONE',  ( 0.000000000000000000, 0.000000000000000000, -1.000000000000000000 ) ) ;
#31910=DIRECTION ( 'NONE',  ( 0.000000000000000000, 0.000000000000000000, 1.000000000000000000 ) ) ;
#31925=VERTEX_POINT ( 'NONE', #18473 ) ;
#31936=ADVANCED_FACE ( 'NONE', ( #13791 ), #8552, .T. ) ;
#31938=DIRECTION ( 'NONE',  ( 0.000000000000000000, 0.000000000000000000, 1.000000000000000000 ) ) ;
#31987=ORIENTED_EDGE ( 'NONE', *, *, #33311, .F. ) ;
#32006=CARTESIAN_POINT ( 'NONE',  ( 9.714451465470119729E-14, 0.9999999999999870104, -44.50000000000000000 ) ) ;
#32047=FACE_OUTER_BOUND ( 'NONE', #12076, .T. ) ;
#32072=FACE_OUTER_BOUND ( 'NONE', #22708, .T. ) ;
#32078=SHAPE_REPRESENTATION_RELATIONSHIP ( 'NONE' , 'NONE' ,  #18063, #13375 ) ;
#32108=DIRECTION ( 'NONE',  ( 0.000000000000000000, 0.000000000000000000, -1.000000000000000000 ) ) ;
#32120=ORIENTED_EDGE ( 'NONE', *, *, #14284, .F. ) ;
#32128=EDGE_CURVE ( 'NONE', #1546, #31584, #26007, .T. ) ;
#32133=AXIS2_PLACEMENT_3D ( 'NONE', #20987, #9671, #23345 ) ;
#32152=ORIENTED_EDGE ( 'NONE', *, *, #17197, .T. ) ;
#32185=DIRECTION ( 'NONE',  ( -1.000000000000000000, 0.000000000000000000, 0.000000000000000000 ) ) ;
#32195=ORIENTED_EDGE ( 'NONE', *, *, #3659, .F. ) ;
#32199=LINE ( 'NONE', #18864, #29582 ) ;
#32249=VERTEX_POINT ( 'NONE', #29793 ) ;
#32259=ORIENTED_EDGE ( 'NONE', *, *, #28894, .T. ) ;
#32264=CARTESIAN_POINT ( 'NONE',  ( 3.799999999999999822, 0.000000000000000000, -55.89999999999999858 ) ) ;
#32285=CARTESIAN_POINT ( 'NONE',  ( 4.000000000000000000, 4.898587196589412829E-16, -55.89999999999999858 ) ) ;
#32336=ORIENTED_EDGE ( 'NONE', *, *, #8411, .F. ) ;
#32339=ORIENTED_EDGE ( 'NONE', *, *, #31244, .F. ) ;
#32360=CARTESIAN_POINT ( 'NONE',  ( 0.000000000000000000, 0.000000000000000000, 36.00000000000000000 ) ) ;
#32363=ORIENTED_EDGE ( 'NONE', *, *, #6154, .T. ) ;
#32368=ORIENTED_EDGE ( 'NONE', *, *, #667, .T. ) ;
#32400=CARTESIAN_POINT ( 'NONE',  ( 0.000000000000000000, 0.000000000000000000, 65.00000000000000000 ) ) ;
#32460=DIRECTION ( 'NONE',  ( 0.000000000000000000, 0.000000000000000000, 1.000000000000000000 ) ) ;
#32465=DIRECTION ( 'NONE',  ( 1.000000000000000000, -1.110223024625156540E-16, 0.000000000000000000 ) ) ;
#32469=DIRECTION ( 'NONE',  ( -0.000000000000000000, 0.000000000000000000, -1.000000000000000000 ) ) ;
#32476=DIRECTION ( 'NONE',  ( -1.000000000000000000, 0.000000000000000000, 0.000000000000000000 ) ) ;
#32488=CIRCLE ( 'NONE', #24456, 4.000000000000000000 ) ;
#32517=CIRCLE ( 'NONE', #16980, 3.799999999999999822 ) ;
#32524=DIRECTION ( 'NONE',  ( 0.000000000000000000, 0.000000000000000000, 1.000000000000000000 ) ) ;
#32529=DIRECTION ( 'NONE',  ( 0.000000000000000000, 0.000000000000000000, 1.000000000000000000 ) ) ;
#32575=ORIENTED_EDGE ( 'NONE', *, *, #12873, .F. ) ;
#32583=CIRCLE ( 'NONE', #29156, 4.000000000000000000 ) ;
#32591=ADVANCED_FACE ( 'NONE', ( #33848, #64 ), #10879, .T. ) ;
#32627=EDGE_CURVE ( 'NONE', #26146, #33746, #21802, .T. ) ;
#32629=LINE ( 'NONE', #21452, #18553 ) ;
#32641=AXIS2_PLACEMENT_3D ( 'NONE', #27478, #16460, #10375 ) ;
#32659=AXIS2_PLACEMENT_3D ( 'NONE', #29177, #4527, #15456 ) ;
#32664=VECTOR ( 'NONE', #19043, 1000.000000000000000 ) ;
#32674=DIRECTION ( 'NONE',  ( 0.000000000000000000, 0.000000000000000000, 1.000000000000000000 ) ) ;
#32725=ORIENTED_EDGE ( 'NONE', *, *, #34140, .F. ) ;
#32739=VERTEX_POINT ( 'NONE', #3790 ) ;
#32750=DIRECTION ( 'NONE',  ( -0.000000000000000000, 0.000000000000000000, -1.000000000000000000 ) ) ;
#32808=DIRECTION ( 'NONE',  ( -1.000000000000000000, 1.110223024625156540E-16, 0.000000000000000000 ) ) ;
#32841=AXIS2_PLACEMENT_3D ( 'NONE', #34634, #7602, #29412 ) ;
#32903=CARTESIAN_POINT ( 'NONE',  ( -4.000000000000000000, 0.000000000000000000, 65.00000000000000000 ) ) ;
#32904=ORIENTED_EDGE ( 'NONE', *, *, #5652, .T. ) ;
#32906=EDGE_LOOP ( 'NONE', ( #21208, #18260 ) ) ;
#32949=ORIENTED_EDGE ( 'NONE', *, *, #31321, .T. ) ;
#32969=PLANE ( 'NONE',  #6994 ) ;
#33006=ORIENTED_EDGE ( 'NONE', *, *, #25567, .F. ) ;
#33085=ORIENTED_EDGE ( 'NONE', *, *, #25604, .T. ) ;
#33125=ORIENTED_EDGE ( 'NONE', *, *, #27762, .F. ) ;
#33129=CYLINDRICAL_SURFACE ( 'NONE', #799, 3.799999999999999822 ) ;
#33131=CIRCLE ( 'NONE', #34286, 3.799999999999999822 ) ;
#33146=CIRCLE ( 'NONE', #30823, 4.000000000000000000 ) ;
#33201=ADVANCED_FACE ( 'NONE', ( #21693 ), #2290, .T. ) ;
#33209=VERTEX_POINT ( 'NONE', #7652 ) ;
#33225=ORIENTED_EDGE ( 'NONE', *, *, #28415, .F. ) ;
#33237=LINE ( 'NONE', #33404, #5096 ) ;
#33270=EDGE_CURVE ( 'NONE', #334, #17706, #13676, .T. ) ;
#33311=EDGE_CURVE ( 'NONE', #33746, #17384, #27823, .T. ) ;
#33320=AXIS2_PLACEMENT_3D ( 'NONE', #12603, #23576, #34571 ) ;
#33322=FACE_OUTER_BOUND ( 'NONE', #28000, .T. ) ;
#33348=ORIENTED_EDGE ( 'NONE', *, *, #27347, .T. ) ;
#33404=CARTESIAN_POINT ( 'NONE',  ( 3.872983346207517386, -1.000000000000028644, 65.00000000000000000 ) ) ;
#33416=VERTEX_POINT ( 'NONE', #27652 ) ;
#33456=AXIS2_PLACEMENT_3D ( 'NONE', #10802, #19063, #21759 ) ;
#33491=DIRECTION ( 'NONE',  ( -1.000000000000000000, 0.000000000000000000, 0.000000000000000000 ) ) ;
#33507=ORIENTED_EDGE ( 'NONE', *, *, #30607, .T. ) ;
#33549=VERTEX_POINT ( 'NONE', #16363 ) ;
#33559=DIRECTION ( 'NONE',  ( 0.000000000000000000, 0.000000000000000000, -1.000000000000000000 ) ) ;
#33565=ORIENTED_EDGE ( 'NONE', *, *, #10734, .F. ) ;
#33610=AXIS2_PLACEMENT_3D ( 'NONE', #22791, #28921, #34507 ) ;
#33643=DIRECTION ( 'NONE',  ( 0.000000000000000000, 0.000000000000000000, -1.000000000000000000 ) ) ;
#33644=EDGE_CURVE ( 'NONE', #10690, #21576, #11510, .T. ) ;
#33666=AXIS2_PLACEMENT_3D ( 'NONE', #3669, #27970, #11581 ) ;
#33713=ADVANCED_FACE ( 'NONE', ( #3243 ), #14206, .F. ) ;
#33721=PLANE ( 'NONE',  #33666 ) ;
#33731=DIRECTION ( 'NONE',  ( -1.000000000000000000, 0.000000000000000000, 0.000000000000000000 ) ) ;
#33732=FACE_BOUND ( 'NONE', #94, .T. ) ;
#33746=VERTEX_POINT ( 'NONE', #9338 ) ;
#33747=ORIENTED_EDGE ( 'NONE', *, *, #22461, .T. ) ;
#33749=EDGE_LOOP ( 'NONE', ( #13169, #20748, #35144, #12617 ) ) ;
#33785=AXIS2_PLACEMENT_3D ( 'NONE', #17272, #30457, #31149 ) ;
#33789=FACE_OUTER_BOUND ( 'NONE', #1185, .T. ) ;
#33803=VECTOR ( 'NONE', #35, 1000.000000000000000 ) ;
#33805=ORIENTED_EDGE ( 'NONE', *, *, #25365, .F. ) ;
#33807=FACE_OUTER_BOUND ( 'NONE', #30967, .T. ) ;
#33813=CARTESIAN_POINT ( 'NONE',  ( -3.799999999999999822, 4.653657836759942730E-16, 60.90000000000001279 ) ) ;
#33821=LINE ( 'NONE', #28772, #17804 ) ;
#33845=ORIENTED_EDGE ( 'NONE', *, *, #5962, .T. ) ;
#33848=FACE_OUTER_BOUND ( 'NONE', #5708, .T. ) ;
#33864=CARTESIAN_POINT ( 'NONE',  ( 5.400000000000085620, -1.000000000000049516, -52.50000000000000000 ) ) ;
#33868=CARTESIAN_POINT ( 'NONE',  ( 3.872983346207489852, 0.9999999999999522604, 55.00000000000000711 ) ) ;
#33886=ORIENTED_EDGE ( 'NONE', *, *, #925, .T. ) ;
#33890=EDGE_CURVE ( 'NONE', #33746, #26146, #22293, .T. ) ;
#33895=ORIENTED_EDGE ( 'NONE', *, *, #1708, .T. ) ;
#33960=FACE_OUTER_BOUND ( 'NONE', #20129, .T. ) ;
#33965=CARTESIAN_POINT ( 'NONE',  ( 3.872983346207489852, 0.9999999999999522604, 65.00000000000000000 ) ) ;
#34005=LINE ( 'NONE', #23363, #30187 ) ;
#34016=DIRECTION ( 'NONE',  ( 0.000000000000000000, 0.000000000000000000, 1.000000000000000000 ) ) ;
#34043=EDGE_LOOP ( 'NONE', ( #1422, #34217, #33886, #34678, #3649, #32195, #27106, #28529 ) ) ;
#34098=DIRECTION ( 'NONE',  ( 0.000000000000000000, 0.000000000000000000, 1.000000000000000000 ) ) ;
#34137=FACE_BOUND ( 'NONE', #26751, .T. ) ;
#34140=EDGE_CURVE ( 'NONE', #10539, #1825, #28041, .T. ) ;
#34149=CYLINDRICAL_SURFACE ( 'NONE', #33610, 4.000000000000000000 ) ;
#34209=AXIS2_PLACEMENT_3D ( 'NONE', #27594, #8295, #21806 ) ;
#34210=EDGE_CURVE ( 'NONE', #18156, #2615, #3917, .T. ) ;
#34217=ORIENTED_EDGE ( 'NONE', *, *, #17189, .T. ) ;
#34226=MANIFOLD_SOLID_BREP ( 'Boss-Extrude2', #27337 ) ;
#34278=AXIS2_PLACEMENT_3D ( 'NONE', #20422, #9465, #12534 ) ;
#34286=AXIS2_PLACEMENT_3D ( 'NONE', #3339, #33559, #9074 ) ;
#34305=AXIS2_PLACEMENT_3D ( 'NONE', #17875, #4224, #17701 ) ;
#34307=ORIENTED_EDGE ( 'NONE', *, *, #23155, .T. ) ;
#34361=DIRECTION ( 'NONE',  ( 0.000000000000000000, 0.000000000000000000, 1.000000000000000000 ) ) ;
#34411=CARTESIAN_POINT ( 'NONE',  ( 0.000000000000000000, 0.000000000000000000, 35.10000000000000142 ) ) ;
#34433=EDGE_LOOP ( 'NONE', ( #9244, #23936 ) ) ;
#34446=LINE ( 'NONE', #21080, #20057 ) ;
#34452=DIRECTION ( 'NONE',  ( -1.000000000000000000, 0.000000000000000000, 0.000000000000000000 ) ) ;
#34459=CARTESIAN_POINT ( 'NONE',  ( 3.799999999999999822, 0.000000000000000000, -32.00000000000000000 ) ) ;
#34496=LINE ( 'NONE', #17548, #8911 ) ;
#34507=DIRECTION ( 'NONE',  ( -1.000000000000000000, 0.000000000000000000, 0.000000000000000000 ) ) ;
#34542=AXIS2_PLACEMENT_3D ( 'NONE', #12709, #10366, #7298 ) ;
#34571=DIRECTION ( 'NONE',  ( -1.000000000000000000, 0.000000000000000000, 0.000000000000000000 ) ) ;
#34577=LINE ( 'NONE', #15997, #1608 ) ;
#34581=VERTEX_POINT ( 'NONE', #19678 ) ;
#34592=EDGE_CURVE ( 'NONE', #11649, #19295, #33131, .T. ) ;
#34605=ORIENTED_EDGE ( 'NONE', *, *, #17197, .F. ) ;
#34616=LINE ( 'NONE', #12106, #18361 ) ;
#34626=VERTEX_POINT ( 'NONE', #14636 ) ;
#34634=CARTESIAN_POINT ( 'NONE',  ( 0.000000000000000000, 0.000000000000000000, -44.50000000000000000 ) ) ;
#34678=ORIENTED_EDGE ( 'NONE', *, *, #5652, .F. ) ;
#34685=FILL_AREA_STYLE_COLOUR ( '', #11335 ) ;
#34691=ORIENTED_EDGE ( 'NONE', *, *, #5498, .F. ) ;
#34703=CARTESIAN_POINT ( 'NONE',  ( 0.000000000000000000, 0.000000000000000000, -32.00000000000000000 ) ) ;
#34754=DIRECTION ( 'NONE',  ( 1.000000000000000000, 0.000000000000000000, 0.000000000000000000 ) ) ;
#34777=ORIENTED_EDGE ( 'NONE', *, *, #7750, .T. ) ;
#34781=( NAMED_UNIT ( * ) SI_UNIT ( $, .STERADIAN. ) SOLID_ANGLE_UNIT ( ) );
#34786=EDGE_CURVE ( 'NONE', #17651, #1850, #29051, .T. ) ;
#34791=EDGE_CURVE ( 'NONE', #31889, #24508, #8415, .T. ) ;
#34819=VECTOR ( 'NONE', #3018, 1000.000000000000000 ) ;
#34838=EDGE_CURVE ( 'NONE', #28168, #5282, #32583, .T. ) ;
#34873=EDGE_CURVE ( 'NONE', #3282, #35360, #26904, .T. ) ;
#34919=ORIENTED_EDGE ( 'NONE', *, *, #4281, .T. ) ;
#34930=ORIENTED_EDGE ( 'NONE', *, *, #29694, .F. ) ;
#34953=CARTESIAN_POINT ( 'NONE',  ( 0.000000000000000000, 0.000000000000000000, -44.50000000000000000 ) ) ;
#35047=CARTESIAN_POINT ( 'NONE',  ( 3.872983346207489852, 0.9999999999999522604, -32.00000000000000000 ) ) ;
#35060=EDGE_CURVE ( 'NONE', #35360, #18475, #4431, .T. ) ;
#35092=VERTEX_POINT ( 'NONE', #1115 ) ;
#35129=DIRECTION ( 'NONE',  ( 1.000000000000000000, 0.000000000000000000, 0.000000000000000000 ) ) ;
#35138=CARTESIAN_POINT ( 'NONE',  ( -3.799999999999999822, 4.653657836759942730E-16, -43.60000000000000142 ) ) ;
#35144=ORIENTED_EDGE ( 'NONE', *, *, #28355, .T. ) ;
#35161=CARTESIAN_POINT ( 'NONE',  ( 0.000000000000000000, 0.000000000000000000, 65.00000000000000000 ) ) ;
#35176=APPLICATION_CONTEXT ( 'automotive_design' ) ;
#35195=CARTESIAN_POINT ( 'NONE',  ( 0.000000000000000000, 0.000000000000000000, -55.00000000000000000 ) ) ;
#35210=DIRECTION ( 'NONE',  ( 0.000000000000000000, 0.000000000000000000, -1.000000000000000000 ) ) ;
#35240=LINE ( 'NONE', #7669, #18353 ) ;
#35271=DIRECTION ( 'NONE',  ( 0.000000000000000000, 1.000000000000000000, 0.000000000000000000 ) ) ;
#35317=CARTESIAN_POINT ( 'NONE',  ( -3.799999999999999822, 4.653657836759942730E-16, -55.00000000000000000 ) ) ;
#35321=ORIENTED_EDGE ( 'NONE', *, *, #21795, .F. ) ;
#35360=VERTEX_POINT ( 'NONE', #35317 ) ;
#35367=CARTESIAN_POINT ( 'NONE',  ( 0.000000000000000000, 0.000000000000000000, 65.00000000000000000 ) ) ;
#35371=FACE_OUTER_BOUND ( 'NONE', #29291, .T. ) ;
#35376=PLANE ( 'NONE',  #31286 ) ;
#35422=DIRECTION ( 'NONE',  ( -1.000000000000000000, 0.000000000000000000, 0.000000000000000000 ) ) ;
#35452=ORIENTED_EDGE ( 'NONE', *, *, #14010, .F. ) ;
#35486=PLANE ( 'NONE',  #5421 ) ;
#35512=DIRECTION ( 'NONE',  ( -1.000000000000000000, 0.000000000000000000, 0.000000000000000000 ) ) ;
#35528=VERTEX_POINT ( 'NONE', #19597 ) ;
#35538=DIRECTION ( 'NONE',  ( -1.000000000000000000, 0.000000000000000000, 0.000000000000000000 ) ) ;
ENDSEC;
END-ISO-10303-21;
